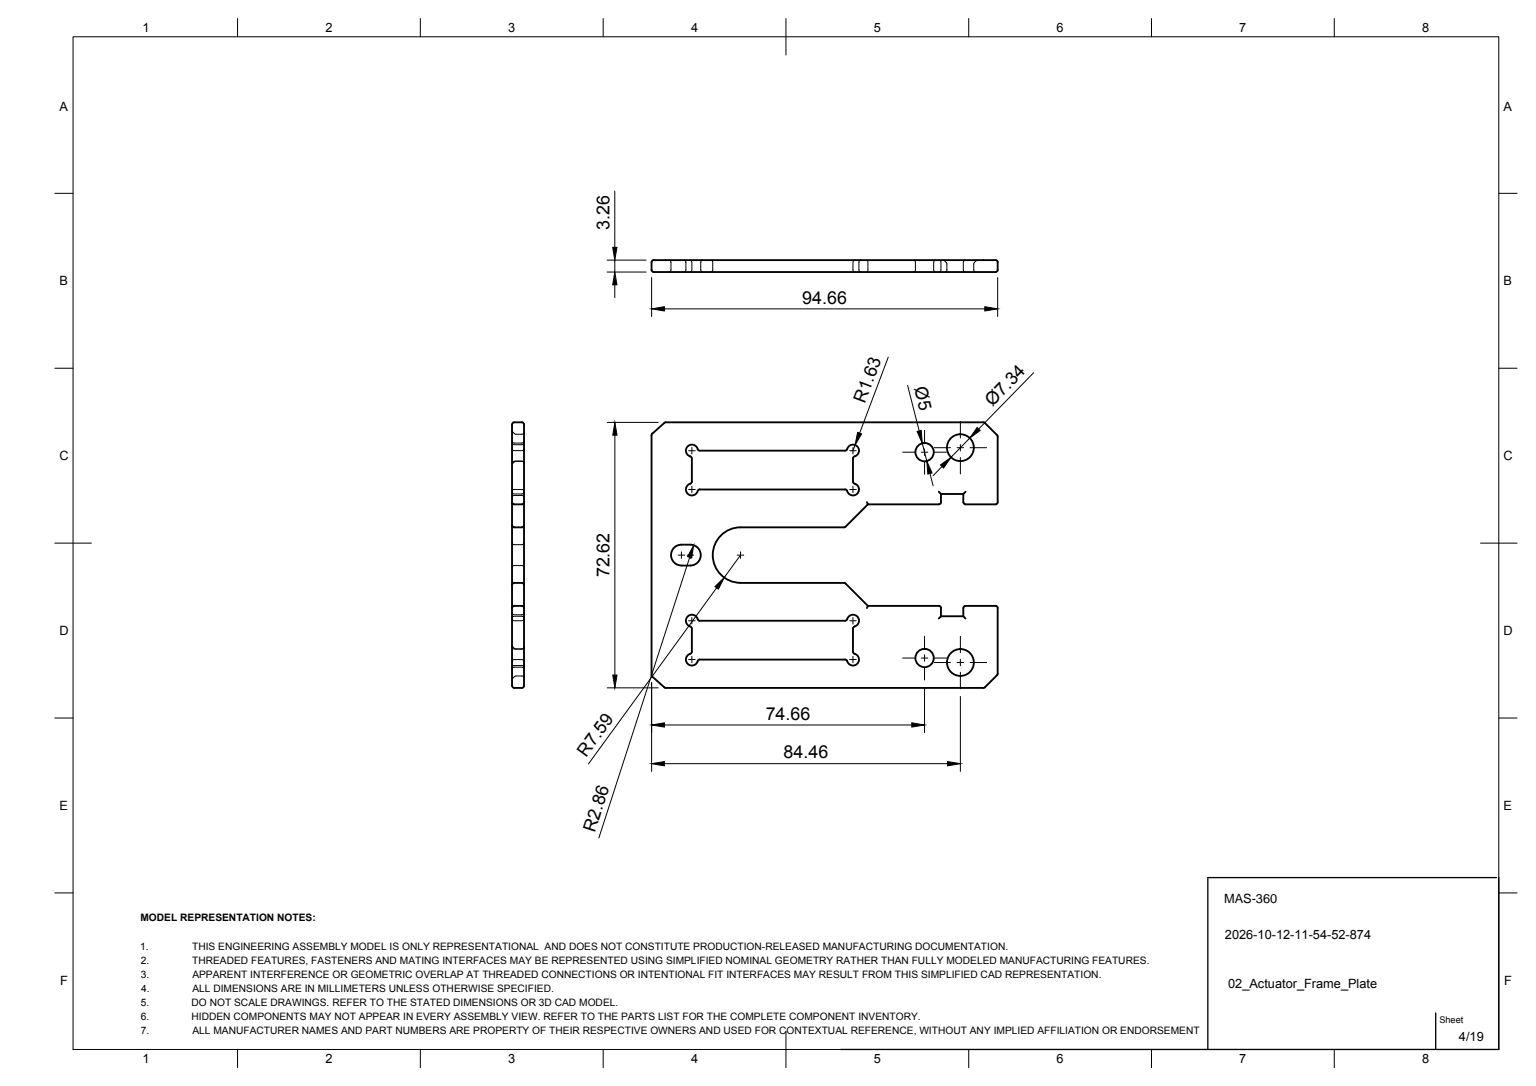
ISO-10303-21;
HEADER;
/* Generated by software containing ST-Developer
 * from STEP Tools, Inc. (www.steptools.com) 
 */

FILE_DESCRIPTION(
/* description */ (''),
/* implementation_level */ '2;1');

FILE_NAME(
/* name */ '02_Actuator_Frame_Plate.step',
/* time_stamp */ '2026-11-04T18:53:29-08:00',
/* author */ (''),
/* organization */ (''),
/* preprocessor_version */ 'ST-DEVELOPER v20.2',
/* originating_system */ 'Autodesk Translation Framework v15.17.0.0',
/* authorisation */ '');

FILE_SCHEMA (('AUTOMOTIVE_DESIGN { 1 0 10303 214 3 1 1 }'));
ENDSEC;

DATA;
#10=MECHANICAL_DESIGN_GEOMETRIC_PRESENTATION_REPRESENTATION('',(#1328),#100031);
#117=SPHERICAL_SURFACE('',#20359,0.6);
#118=SPHERICAL_SURFACE('',#20362,0.6);
#119=SPHERICAL_SURFACE('',#20376,0.6);
#120=SPHERICAL_SURFACE('',#20379,0.6);
#121=SPHERICAL_SURFACE('',#20389,0.6);
#122=SPHERICAL_SURFACE('',#20391,0.6);
#123=SPHERICAL_SURFACE('',#20401,0.6);
#124=SPHERICAL_SURFACE('',#20404,0.6);
#125=SPHERICAL_SURFACE('',#20414,0.6);
#126=SPHERICAL_SURFACE('',#20417,0.6);
#127=SPHERICAL_SURFACE('',#20430,0.6);
#128=SPHERICAL_SURFACE('',#20432,0.6);
#129=SPHERICAL_SURFACE('',#20487,0.6);
#130=SPHERICAL_SURFACE('',#20492,0.6);
#131=SPHERICAL_SURFACE('',#20504,0.6);
#132=SPHERICAL_SURFACE('',#20509,0.600000000000001);
#133=SPHERICAL_SURFACE('',#20513,0.6);
#134=SPHERICAL_SURFACE('',#20518,0.600000000000001);
#135=SPHERICAL_SURFACE('',#20523,0.600000000000001);
#136=SPHERICAL_SURFACE('',#20530,0.6);
#137=SPHERICAL_SURFACE('',#20535,0.6);
#138=SPHERICAL_SURFACE('',#20540,0.6);
#139=SPHERICAL_SURFACE('',#20545,0.6);
#140=SPHERICAL_SURFACE('',#20554,0.6);
#141=SPHERICAL_SURFACE('',#20558,0.6);
#142=SPHERICAL_SURFACE('',#20566,0.6);
#143=SPHERICAL_SURFACE('',#20577,0.6);
#144=SPHERICAL_SURFACE('',#20582,0.6);
#145=SPHERICAL_SURFACE('',#20603,0.600000000000001);
#146=SPHERICAL_SURFACE('',#20608,0.600000000000001);
#147=SPHERICAL_SURFACE('',#20613,0.600000000000001);
#148=SPHERICAL_SURFACE('',#20618,0.600000000000001);
#149=SPHERICAL_SURFACE('',#20627,0.600000000000001);
#150=SPHERICAL_SURFACE('',#20635,0.6);
#151=SPHERICAL_SURFACE('',#20640,0.6);
#152=SPHERICAL_SURFACE('',#20645,0.6);
#153=SPHERICAL_SURFACE('',#20650,0.6);
#154=SPHERICAL_SURFACE('',#20655,0.6);
#155=SPHERICAL_SURFACE('',#20660,0.6);
#156=SPHERICAL_SURFACE('',#20690,0.600000000000001);
#157=SPHERICAL_SURFACE('',#20697,0.6);
#158=SPHERICAL_SURFACE('',#20698,0.6);
#159=SPHERICAL_SURFACE('',#20704,0.6);
#160=SPHERICAL_SURFACE('',#20713,0.600000000000001);
#161=SPHERICAL_SURFACE('',#20716,0.600000000000005);
#162=SPHERICAL_SURFACE('',#20721,0.6);
#163=SPHERICAL_SURFACE('',#20729,0.6);
#164=SPHERICAL_SURFACE('',#20732,0.6);
#165=SPHERICAL_SURFACE('',#20737,0.6);
#166=SPHERICAL_SURFACE('',#20742,0.6);
#167=SPHERICAL_SURFACE('',#20749,0.6);
#168=SPHERICAL_SURFACE('',#20755,0.6);
#169=SPHERICAL_SURFACE('',#20763,0.6);
#170=SPHERICAL_SURFACE('',#20769,0.600000000000001);
#171=SPHERICAL_SURFACE('',#20779,0.600000000000001);
#172=SPHERICAL_SURFACE('',#20788,0.600000000000001);
#173=SPHERICAL_SURFACE('',#20793,0.600000000000001);
#174=SPHERICAL_SURFACE('',#20798,0.600000000000001);
#175=SPHERICAL_SURFACE('',#20810,0.6);
#176=SPHERICAL_SURFACE('',#20815,0.6);
#177=SPHERICAL_SURFACE('',#20820,0.6);
#178=SPHERICAL_SURFACE('',#20825,0.6);
#179=SPHERICAL_SURFACE('',#20830,0.6);
#180=SPHERICAL_SURFACE('',#20832,0.6);
#227=CONICAL_SURFACE('',#20353,4.08,0.785398163397448);
#228=CONICAL_SURFACE('',#20885,4.08,0.785398163397448);
#250=CIRCLE('',#20345,3.84773593128807);
#251=CIRCLE('',#20346,0.6);
#252=CIRCLE('',#20347,3.672);
#253=CIRCLE('',#20348,3.672);
#254=CIRCLE('',#20349,3.84773593128807);
#255=CIRCLE('',#20351,3.672);
#256=CIRCLE('',#20352,3.672);
#257=CIRCLE('',#20354,4.31226406871192);
#258=CIRCLE('',#20355,4.31226406871192);
#259=CIRCLE('',#20357,0.600000000000001);
#260=CIRCLE('',#20358,0.599999999999999);
#261=CIRCLE('',#20360,0.6);
#262=CIRCLE('',#20361,0.599999999999999);
#263=CIRCLE('',#20363,0.599999999999999);
#264=CIRCLE('',#20364,0.6);
#265=CIRCLE('',#20366,0.599999999999999);
#266=CIRCLE('',#20368,1.632);
#267=CIRCLE('',#20369,0.599999999999998);
#268=CIRCLE('',#20370,2.232);
#269=CIRCLE('',#20372,1.632);
#270=CIRCLE('',#20374,0.600000000000001);
#271=CIRCLE('',#20375,0.599999999999998);
#272=CIRCLE('',#20377,0.6);
#273=CIRCLE('',#20378,0.599999999999999);
#274=CIRCLE('',#20380,0.6);
#275=CIRCLE('',#20382,2.232);
#276=CIRCLE('',#20383,0.6);
#277=CIRCLE('',#20384,1.632);
#278=CIRCLE('',#20387,0.600000000000001);
#279=CIRCLE('',#20388,0.599999999999998);
#280=CIRCLE('',#20390,0.599999999999999);
#281=CIRCLE('',#20392,0.599999999999999);
#282=CIRCLE('',#20393,0.6);
#283=CIRCLE('',#20395,0.599999999999999);
#284=CIRCLE('',#20397,1.632);
#285=CIRCLE('',#20399,0.600000000000001);
#286=CIRCLE('',#20400,0.600000000000003);
#287=CIRCLE('',#20402,0.6);
#288=CIRCLE('',#20403,0.599999999999999);
#289=CIRCLE('',#20405,0.6);
#290=CIRCLE('',#20407,2.232);
#291=CIRCLE('',#20408,0.600000000000001);
#292=CIRCLE('',#20409,1.632);
#293=CIRCLE('',#20412,0.600000000000001);
#294=CIRCLE('',#20413,0.600000000000003);
#295=CIRCLE('',#20415,0.6);
#296=CIRCLE('',#20416,0.6);
#297=CIRCLE('',#20418,0.6);
#298=CIRCLE('',#20419,0.6);
#299=CIRCLE('',#20421,2.232);
#300=CIRCLE('',#20422,0.6);
#301=CIRCLE('',#20423,1.632);
#302=CIRCLE('',#20425,0.6);
#303=CIRCLE('',#20428,0.599999999999996);
#304=CIRCLE('',#20429,0.599999999999999);
#305=CIRCLE('',#20431,0.599999999999999);
#306=CIRCLE('',#20433,0.599999999999999);
#307=CIRCLE('',#20434,0.6);
#308=CIRCLE('',#20436,0.599999999999999);
#309=CIRCLE('',#20438,1.632);
#310=CIRCLE('',#20440,3.1);
#311=CIRCLE('',#20441,0.6);
#312=CIRCLE('',#20442,2.5);
#313=CIRCLE('',#20443,2.5);
#314=CIRCLE('',#20445,8.1888);
#315=CIRCLE('',#20446,4.272);
#316=CIRCLE('',#20447,3.456);
#317=CIRCLE('',#20448,3.456);
#318=CIRCLE('',#20449,2.232);
#319=CIRCLE('',#20450,2.232);
#320=CIRCLE('',#20451,2.232);
#321=CIRCLE('',#20452,2.232);
#322=CIRCLE('',#20453,3.1);
#323=CIRCLE('',#20454,2.232);
#324=CIRCLE('',#20455,2.232);
#325=CIRCLE('',#20456,2.232);
#326=CIRCLE('',#20457,2.232);
#327=CIRCLE('',#20458,4.272);
#328=CIRCLE('',#20460,2.5);
#329=CIRCLE('',#20461,2.5);
#330=CIRCLE('',#20463,0.6);
#331=CIRCLE('',#20464,3.672);
#332=CIRCLE('',#20465,3.672);
#333=CIRCLE('',#20467,3.672);
#334=CIRCLE('',#20468,3.672);
#335=CIRCLE('',#20470,0.6);
#336=CIRCLE('',#20472,0.600000000000005);
#337=CIRCLE('',#20473,0.6);
#338=CIRCLE('',#20475,0.6);
#339=CIRCLE('',#20476,2.856);
#340=CIRCLE('',#20478,0.6);
#341=CIRCLE('',#20480,2.856);
#342=CIRCLE('',#20482,2.856);
#343=CIRCLE('',#20485,0.600000000000001);
#344=CIRCLE('',#20488,0.600000000000001);
#345=CIRCLE('',#20489,0.6);
#346=CIRCLE('',#20490,0.6);
#347=CIRCLE('',#20493,0.600000000000001);
#348=CIRCLE('',#20494,0.6);
#349=CIRCLE('',#20497,0.599999999999998);
#350=CIRCLE('',#20499,0.600000000000001);
#351=CIRCLE('',#20500,1.632);
#352=CIRCLE('',#20503,0.600000000000001);
#353=CIRCLE('',#20505,0.599999999999999);
#354=CIRCLE('',#20506,0.6);
#355=CIRCLE('',#20508,0.600000000000001);
#356=CIRCLE('',#20510,0.600000000000001);
#357=CIRCLE('',#20511,0.600000000000001);
#358=CIRCLE('',#20512,0.599999999999991);
#359=CIRCLE('',#20514,0.600000000000001);
#360=CIRCLE('',#20515,0.6);
#361=CIRCLE('',#20516,0.600000000000003);
#362=CIRCLE('',#20519,0.600000000000001);
#363=CIRCLE('',#20520,0.600000000000001);
#364=CIRCLE('',#20521,0.599999999999996);
#365=CIRCLE('',#20524,0.599999999999996);
#366=CIRCLE('',#20525,0.600000000000001);
#367=CIRCLE('',#20526,0.600000000000001);
#368=CIRCLE('',#20529,0.600000000000001);
#369=CIRCLE('',#20531,0.600000000000003);
#370=CIRCLE('',#20532,0.6);
#371=CIRCLE('',#20534,0.600000000000001);
#372=CIRCLE('',#20536,0.600000000000003);
#373=CIRCLE('',#20537,0.599999999999999);
#374=CIRCLE('',#20539,0.599999999999996);
#375=CIRCLE('',#20541,0.599999999999999);
#376=CIRCLE('',#20542,0.599999999999998);
#377=CIRCLE('',#20544,0.60000000000001);
#378=CIRCLE('',#20546,0.600000000000003);
#379=CIRCLE('',#20547,0.599999999999999);
#380=CIRCLE('',#20552,0.600000000000003);
#381=CIRCLE('',#20555,0.600000000000001);
#382=CIRCLE('',#20556,0.6);
#383=CIRCLE('',#20557,0.600000000000001);
#384=CIRCLE('',#20559,0.6);
#385=CIRCLE('',#20560,0.599999999999999);
#386=CIRCLE('',#20561,0.6);
#387=CIRCLE('',#20564,0.600000000000003);
#388=CIRCLE('',#20565,1.632);
#389=CIRCLE('',#20567,0.600000000000001);
#390=CIRCLE('',#20568,0.6);
#391=CIRCLE('',#20570,0.600000000000005);
#392=CIRCLE('',#20572,1.632);
#393=CIRCLE('',#20573,0.599999999999998);
#394=CIRCLE('',#20578,0.6);
#395=CIRCLE('',#20579,0.6);
#396=CIRCLE('',#20580,0.6);
#397=CIRCLE('',#20583,0.599999999999998);
#398=CIRCLE('',#20585,2.232);
#399=CIRCLE('',#20586,0.6);
#400=CIRCLE('',#20587,1.632);
#401=CIRCLE('',#20589,0.599999999999999);
#402=CIRCLE('',#20592,0.600000000000004);
#403=CIRCLE('',#20595,0.600000000000001);
#404=CIRCLE('',#20597,0.6);
#405=CIRCLE('',#20598,2.5);
#406=CIRCLE('',#20599,2.5);
#407=CIRCLE('',#20601,2.5);
#408=CIRCLE('',#20602,2.5);
#409=CIRCLE('',#20604,0.600000000000001);
#410=CIRCLE('',#20605,0.600000000000001);
#411=CIRCLE('',#20606,0.599999999999999);
#412=CIRCLE('',#20609,0.599999999999996);
#413=CIRCLE('',#20610,0.600000000000001);
#414=CIRCLE('',#20611,0.599999999999996);
#415=CIRCLE('',#20614,0.599999999999987);
#416=CIRCLE('',#20615,0.600000000000001);
#417=CIRCLE('',#20616,0.600000000000001);
#418=CIRCLE('',#20619,0.600000000000001);
#419=CIRCLE('',#20620,0.600000000000001);
#420=CIRCLE('',#20621,0.600000000000001);
#421=CIRCLE('',#20628,0.600000000000005);
#422=CIRCLE('',#20629,0.600000000000001);
#423=CIRCLE('',#20630,0.600000000000001);
#424=CIRCLE('',#20634,0.600000000000001);
#425=CIRCLE('',#20636,0.599999999999999);
#426=CIRCLE('',#20637,0.599999999999999);
#427=CIRCLE('',#20639,0.600000000000001);
#428=CIRCLE('',#20641,0.600000000000003);
#429=CIRCLE('',#20642,0.599999999999999);
#430=CIRCLE('',#20644,0.600000000000001);
#431=CIRCLE('',#20646,0.599999999999999);
#432=CIRCLE('',#20647,0.599999999999999);
#433=CIRCLE('',#20649,0.599999999999996);
#434=CIRCLE('',#20651,0.599999999999999);
#435=CIRCLE('',#20652,0.600000000000001);
#436=CIRCLE('',#20654,0.599999999999996);
#437=CIRCLE('',#20656,0.600000000000003);
#438=CIRCLE('',#20657,0.599999999999999);
#439=CIRCLE('',#20659,0.600000000000001);
#440=CIRCLE('',#20661,0.599999999999999);
#441=CIRCLE('',#20678,3.1);
#442=CIRCLE('',#20679,0.6);
#443=CIRCLE('',#20681,8.1888);
#444=CIRCLE('',#20682,2.232);
#445=CIRCLE('',#20683,2.232);
#446=CIRCLE('',#20684,2.232);
#447=CIRCLE('',#20685,3.456);
#448=CIRCLE('',#20686,3.456);
#449=CIRCLE('',#20687,4.73652813742386);
#450=CIRCLE('',#20688,4.73652813742386);
#451=CIRCLE('',#20689,3.1);
#452=CIRCLE('',#20691,0.600000000000001);
#453=CIRCLE('',#20693,0.600000000000001);
#454=CIRCLE('',#20696,0.600000000000003);
#455=CIRCLE('',#20705,0.600000000000001);
#456=CIRCLE('',#20706,0.600000000000003);
#457=CIRCLE('',#20707,0.6);
#458=CIRCLE('',#20714,0.599999999999999);
#459=CIRCLE('',#20715,0.600000000000001);
#460=CIRCLE('',#20717,0.600000000000001);
#461=CIRCLE('',#20718,0.600000000000005);
#462=CIRCLE('',#20719,0.599999999999998);
#463=CIRCLE('',#20722,0.599999999999998);
#464=CIRCLE('',#20723,0.599999999999999);
#465=CIRCLE('',#20724,0.599999999999999);
#466=CIRCLE('',#20726,1.632);
#467=CIRCLE('',#20728,0.599999999999998);
#468=CIRCLE('',#20730,0.6);
#469=CIRCLE('',#20731,0.599999999999999);
#470=CIRCLE('',#20733,0.6);
#471=CIRCLE('',#20734,0.599999999999999);
#472=CIRCLE('',#20735,0.6);
#473=CIRCLE('',#20738,0.6);
#474=CIRCLE('',#20740,1.632);
#475=CIRCLE('',#20743,0.599999999999998);
#476=CIRCLE('',#20744,0.6);
#477=CIRCLE('',#20747,1.632);
#478=CIRCLE('',#20748,0.600000000000003);
#479=CIRCLE('',#20750,0.600000000000001);
#480=CIRCLE('',#20751,0.599999999999999);
#481=CIRCLE('',#20753,0.6);
#482=CIRCLE('',#20754,1.632);
#483=CIRCLE('',#20756,0.6);
#484=CIRCLE('',#20757,0.599999999999999);
#485=CIRCLE('',#20758,0.6);
#486=CIRCLE('',#20762,0.600000000000003);
#487=CIRCLE('',#20764,0.599999999999999);
#488=CIRCLE('',#20768,0.599999999999999);
#489=CIRCLE('',#20770,0.600000000000001);
#490=CIRCLE('',#20771,0.600000000000001);
#491=CIRCLE('',#20772,0.599999999999999);
#492=CIRCLE('',#20774,0.600000000000001);
#493=CIRCLE('',#20775,7.5888);
#494=CIRCLE('',#20780,0.600000000000001);
#495=CIRCLE('',#20781,0.600000000000001);
#496=CIRCLE('',#20782,0.600000000000001);
#497=CIRCLE('',#20789,0.600000000000001);
#498=CIRCLE('',#20790,0.600000000000001);
#499=CIRCLE('',#20791,0.600000000000001);
#500=CIRCLE('',#20794,0.600000000000001);
#501=CIRCLE('',#20795,0.600000000000001);
#502=CIRCLE('',#20796,0.599999999999996);
#503=CIRCLE('',#20799,0.599999999999996);
#504=CIRCLE('',#20800,0.600000000000001);
#505=CIRCLE('',#20801,0.599999999999999);
#506=CIRCLE('',#20805,0.599999999999999);
#507=CIRCLE('',#20807,0.600000000000001);
#508=CIRCLE('',#20809,0.599999999999996);
#509=CIRCLE('',#20811,0.599999999999999);
#510=CIRCLE('',#20812,0.599999999999999);
#511=CIRCLE('',#20814,0.600000000000001);
#512=CIRCLE('',#20816,0.599999999999999);
#513=CIRCLE('',#20817,0.600000000000003);
#514=CIRCLE('',#20819,0.600000000000001);
#515=CIRCLE('',#20821,0.599999999999999);
#516=CIRCLE('',#20822,0.599999999999999);
#517=CIRCLE('',#20824,0.599999999999999);
#518=CIRCLE('',#20826,0.599999999999999);
#519=CIRCLE('',#20827,0.6);
#520=CIRCLE('',#20829,0.600000000000001);
#521=CIRCLE('',#20831,0.599999999999999);
#522=CIRCLE('',#20833,0.6);
#523=CIRCLE('',#20835,0.600000000000001);
#524=CIRCLE('',#20855,0.600000000000001);
#525=CIRCLE('',#20857,7.5888);
#526=CIRCLE('',#20863,1.632);
#527=CIRCLE('',#20868,0.6);
#528=CIRCLE('',#20870,0.600000000000001);
#529=CIRCLE('',#20871,0.6);
#530=CIRCLE('',#20873,0.6);
#531=CIRCLE('',#20874,2.856);
#532=CIRCLE('',#20876,0.6);
#533=CIRCLE('',#20880,0.6);
#534=CIRCLE('',#20882,4.31226406871192);
#535=CIRCLE('',#20883,0.6);
#536=CIRCLE('',#20884,4.31226406871192);
#537=CIRCLE('',#20886,3.84773593128807);
#538=CIRCLE('',#20887,3.84773593128807);
#539=CIRCLE('',#20889,0.6);
#1183=TOROIDAL_SURFACE('',#20344,4.272,0.6);
#1184=TOROIDAL_SURFACE('',#20367,2.232,0.6);
#1185=TOROIDAL_SURFACE('',#20381,2.232,0.6);
#1186=TOROIDAL_SURFACE('',#20406,2.232,0.6);
#1187=TOROIDAL_SURFACE('',#20420,2.232,0.6);
#1188=TOROIDAL_SURFACE('',#20439,3.1,0.6);
#1189=TOROIDAL_SURFACE('',#20462,4.272,0.6);
#1190=TOROIDAL_SURFACE('',#20469,4.272,0.6);
#1191=TOROIDAL_SURFACE('',#20474,3.456,0.6);
#1192=TOROIDAL_SURFACE('',#20479,3.456,0.6);
#1193=TOROIDAL_SURFACE('',#20486,2.232,0.6);
#1194=TOROIDAL_SURFACE('',#20498,2.232,0.6);
#1195=TOROIDAL_SURFACE('',#20563,2.232,0.6);
#1196=TOROIDAL_SURFACE('',#20571,2.232,0.6);
#1197=TOROIDAL_SURFACE('',#20575,2.232,0.6);
#1198=TOROIDAL_SURFACE('',#20581,2.232,0.6);
#1199=TOROIDAL_SURFACE('',#20584,2.232,0.6);
#1200=TOROIDAL_SURFACE('',#20596,3.1,0.6);
#1201=TOROIDAL_SURFACE('',#20677,3.1,0.6);
#1202=TOROIDAL_SURFACE('',#20725,2.232,0.6);
#1203=TOROIDAL_SURFACE('',#20741,2.232,0.6);
#1204=TOROIDAL_SURFACE('',#20746,2.232,0.6);
#1205=TOROIDAL_SURFACE('',#20752,2.232,0.6);
#1206=TOROIDAL_SURFACE('',#20773,8.1888,0.6);
#1207=TOROIDAL_SURFACE('',#20856,8.1888,0.6);
#1208=TOROIDAL_SURFACE('',#20862,2.232,0.6);
#1209=TOROIDAL_SURFACE('',#20867,3.1,0.6);
#1210=TOROIDAL_SURFACE('',#20872,3.456,0.6);
#1211=TOROIDAL_SURFACE('',#20877,3.456,0.6);
#1212=TOROIDAL_SURFACE('',#20879,4.73652813742386,0.6);
#1213=TOROIDAL_SURFACE('',#20881,4.73652813742386,0.6);
#1214=TOROIDAL_SURFACE('',#20888,4.272,0.6);
#1292=SHAPE_REPRESENTATION_RELATIONSHIP('SRR','None',#100102,#1310);
#1310=ADVANCED_BREP_SHAPE_REPRESENTATION('',(#1346),#100014);
#1328=STYLED_ITEM('',(#100201),#1346);
#1346=MANIFOLD_SOLID_BREP('Body1',#20118);
#1364=PLANE('',#20385);
#1365=PLANE('',#20410);
#1366=PLANE('',#20426);
#1367=PLANE('',#20444);
#1368=PLANE('',#20483);
#1369=PLANE('',#20495);
#1370=PLANE('',#20548);
#1371=PLANE('',#20549);
#1372=PLANE('',#20553);
#1373=PLANE('',#20590);
#1374=PLANE('',#20662);
#1375=PLANE('',#20665);
#1376=PLANE('',#20669);
#1377=PLANE('',#20670);
#1378=PLANE('',#20671);
#1379=PLANE('',#20676);
#1380=PLANE('',#20680);
#1381=PLANE('',#20700);
#1382=PLANE('',#20709);
#1383=PLANE('',#20710);
#1384=PLANE('',#20711);
#1385=PLANE('',#20765);
#1386=PLANE('',#20838);
#1387=PLANE('',#20839);
#1388=PLANE('',#20843);
#1389=PLANE('',#20844);
#1390=PLANE('',#20845);
#1391=PLANE('',#20848);
#1392=PLANE('',#20850);
#1393=PLANE('',#20852);
#1394=PLANE('',#20858);
#1395=PLANE('',#20860);
#1396=PLANE('',#20866);
#1397=PLANE('',#20890);
#1398=PLANE('',#20891);
#1703=FACE_BOUND('',#6316,.T.);
#1704=FACE_BOUND('',#6317,.T.);
#1705=FACE_BOUND('',#6318,.T.);
#1706=FACE_BOUND('',#6319,.T.);
#1707=FACE_BOUND('',#6320,.T.);
#1708=FACE_BOUND('',#6321,.T.);
#1709=FACE_BOUND('',#6322,.T.);
#1710=FACE_BOUND('',#6424,.T.);
#1711=FACE_BOUND('',#6425,.T.);
#1712=FACE_BOUND('',#6426,.T.);
#1713=FACE_BOUND('',#6427,.T.);
#1714=FACE_BOUND('',#6428,.T.);
#1715=FACE_BOUND('',#6429,.T.);
#1716=FACE_BOUND('',#6430,.T.);
#1813=ELLIPSE('',#20502,0.649435320175436,0.6);
#1814=ELLIPSE('',#20624,0.848528137423857,0.6);
#1815=ELLIPSE('',#20626,0.848528137423857,0.6);
#1816=ELLIPSE('',#20668,0.848528137423857,0.6);
#1817=ELLIPSE('',#20673,0.848528137423857,0.6);
#1818=ELLIPSE('',#20675,0.649435320175435,0.6);
#1819=ELLIPSE('',#20778,0.649435320175437,0.6);
#1820=ELLIPSE('',#20785,0.848528137423857,0.6);
#1821=ELLIPSE('',#20787,0.848528137423857,0.6);
#1822=ELLIPSE('',#20837,0.649435320175436,0.6);
#1823=ELLIPSE('',#20842,0.848528137423857,0.6);
#1824=ELLIPSE('',#20847,0.848528137423857,0.6);
#2070=LINE('',#59081,#3357);
#2071=LINE('',#59084,#3358);
#2072=LINE('',#59093,#3359);
#2073=LINE('',#59096,#3360);
#2074=LINE('',#59107,#3361);
#2075=LINE('',#59110,#3362);
#2076=LINE('',#59120,#3363);
#2077=LINE('',#59125,#3364);
#2078=LINE('',#59128,#3365);
#2079=LINE('',#59142,#3366);
#2080=LINE('',#59147,#3367);
#2081=LINE('',#59150,#3368);
#2082=LINE('',#59159,#3369);
#2083=LINE('',#59162,#3370);
#2084=LINE('',#59169,#3371);
#2085=LINE('',#59172,#3372);
#2086=LINE('',#59186,#3373);
#2087=LINE('',#59192,#3374);
#2088=LINE('',#59195,#3375);
#2089=LINE('',#59212,#3376);
#2090=LINE('',#59215,#3377);
#2091=LINE('',#59218,#3378);
#2092=LINE('',#59219,#3379);
#2093=LINE('',#59224,#3380);
#2094=LINE('',#59227,#3381);
#2095=LINE('',#59236,#3382);
#2096=LINE('',#59239,#3383);
#2097=LINE('',#59253,#3384);
#2098=LINE('',#59255,#3385);
#2099=LINE('',#59257,#3386);
#2100=LINE('',#59259,#3387);
#2101=LINE('',#59261,#3388);
#2102=LINE('',#59263,#3389);
#2103=LINE('',#59265,#3390);
#2104=LINE('',#59267,#3391);
#2105=LINE('',#59269,#3392);
#2106=LINE('',#59271,#3393);
#2107=LINE('',#59273,#3394);
#2108=LINE('',#59275,#3395);
#2109=LINE('',#59277,#3396);
#2110=LINE('',#59279,#3397);
#2111=LINE('',#59281,#3398);
#2112=LINE('',#59283,#3399);
#2113=LINE('',#59285,#3400);
#2114=LINE('',#59287,#3401);
#2115=LINE('',#59289,#3402);
#2116=LINE('',#59291,#3403);
#2117=LINE('',#59293,#3404);
#2118=LINE('',#59295,#3405);
#2119=LINE('',#59298,#3406);
#2120=LINE('',#59303,#3407);
#2121=LINE('',#59307,#3408);
#2122=LINE('',#59310,#3409);
#2123=LINE('',#59314,#3410);
#2124=LINE('',#59318,#3411);
#2125=LINE('',#59321,#3412);
#2126=LINE('',#59329,#3413);
#2127=LINE('',#59331,#3414);
#2128=LINE('',#59333,#3415);
#2129=LINE('',#59336,#3416);
#2130=LINE('',#59341,#3417);
#2131=LINE('',#59353,#3418);
#2132=LINE('',#59363,#3419);
#2133=LINE('',#59372,#3420);
#2134=LINE('',#59377,#3421);
#2135=LINE('',#59380,#3422);
#2136=LINE('',#59383,#3423);
#2137=LINE('',#59384,#3424);
#2138=LINE('',#59387,#3425);
#2139=LINE('',#59401,#3426);
#2140=LINE('',#59404,#3427);
#2141=LINE('',#59415,#3428);
#2142=LINE('',#59423,#3429);
#2143=LINE('',#59437,#3430);
#2144=LINE('',#59445,#3431);
#2145=LINE('',#59453,#3432);
#2146=LINE('',#59457,#3433);
#2147=LINE('',#59466,#3434);
#2148=LINE('',#59467,#3435);
#2149=LINE('',#59476,#3436);
#2150=LINE('',#59477,#3437);
#2151=LINE('',#59486,#3438);
#2152=LINE('',#59487,#3439);
#2153=LINE('',#59493,#3440);
#2154=LINE('',#59495,#3441);
#2155=LINE('',#59497,#3442);
#2156=LINE('',#59500,#3443);
#2157=LINE('',#59503,#3444);
#2158=LINE('',#59505,#3445);
#2159=LINE('',#59520,#3446);
#2160=LINE('',#59521,#3447);
#2161=LINE('',#59533,#3448);
#2162=LINE('',#59557,#3449);
#2163=LINE('',#59559,#3450);
#2164=LINE('',#59561,#3451);
#2165=LINE('',#59563,#3452);
#2166=LINE('',#59568,#3453);
#2167=LINE('',#59578,#3454);
#2168=LINE('',#59589,#3455);
#2169=LINE('',#59597,#3456);
#2170=LINE('',#59605,#3457);
#2171=LINE('',#59613,#3458);
#2172=LINE('',#59616,#3459);
#2173=LINE('',#59621,#3460);
#2174=LINE('',#59629,#3461);
#2175=LINE('',#59631,#3462);
#2176=LINE('',#59636,#3463);
#2177=LINE('',#59637,#3464);
#2178=LINE('',#59646,#3465);
#2179=LINE('',#59647,#3466);
#2180=LINE('',#59656,#3467);
#2181=LINE('',#59657,#3468);
#2182=LINE('',#59666,#3469);
#2183=LINE('',#59667,#3470);
#2184=LINE('',#59676,#3471);
#2185=LINE('',#59677,#3472);
#2186=LINE('',#59684,#3473);
#2187=LINE('',#59689,#3474);
#2188=LINE('',#59691,#3475);
#2189=LINE('',#59692,#3476);
#2190=LINE('',#59694,#3477);
#2191=LINE('',#59696,#3478);
#2192=LINE('',#59698,#3479);
#2193=LINE('',#59701,#3480);
#2194=LINE('',#59704,#3481);
#2195=LINE('',#59706,#3482);
#2196=LINE('',#59709,#3483);
#2197=LINE('',#59710,#3484);
#2198=LINE('',#59712,#3485);
#2199=LINE('',#59715,#3486);
#2200=LINE('',#59719,#3487);
#2201=LINE('',#59722,#3488);
#2202=LINE('',#59724,#3489);
#2203=LINE('',#59731,#3490);
#2204=LINE('',#59733,#3491);
#2205=LINE('',#59737,#3492);
#2206=LINE('',#59739,#3493);
#2207=LINE('',#59741,#3494);
#2208=LINE('',#59743,#3495);
#2209=LINE('',#59745,#3496);
#2210=LINE('',#59747,#3497);
#2211=LINE('',#59749,#3498);
#2212=LINE('',#59751,#3499);
#2213=LINE('',#59753,#3500);
#2214=LINE('',#59754,#3501);
#2215=LINE('',#59755,#3502);
#2216=LINE('',#59756,#3503);
#2217=LINE('',#59757,#3504);
#2218=LINE('',#59761,#3505);
#2219=LINE('',#59765,#3506);
#2220=LINE('',#59769,#3507);
#2221=LINE('',#59773,#3508);
#2222=LINE('',#59777,#3509);
#2223=LINE('',#59787,#3510);
#2224=LINE('',#59789,#3511);
#2225=LINE('',#59791,#3512);
#2226=LINE('',#59793,#3513);
#2227=LINE('',#59800,#3514);
#2228=LINE('',#59809,#3515);
#2229=LINE('',#59813,#3516);
#2230=LINE('',#59815,#3517);
#2231=LINE('',#59827,#3518);
#2232=LINE('',#59840,#3519);
#2233=LINE('',#59841,#3520);
#2234=LINE('',#59852,#3521);
#2235=LINE('',#59853,#3522);
#2236=LINE('',#59864,#3523);
#2237=LINE('',#59884,#3524);
#2238=LINE('',#59885,#3525);
#2239=LINE('',#59887,#3526);
#2240=LINE('',#59889,#3527);
#2241=LINE('',#59892,#3528);
#2242=LINE('',#59896,#3529);
#2243=LINE('',#59901,#3530);
#2244=LINE('',#59913,#3531);
#2245=LINE('',#59916,#3532);
#2246=LINE('',#59925,#3533);
#2247=LINE('',#59928,#3534);
#2248=LINE('',#59933,#3535);
#2249=LINE('',#59941,#3536);
#2250=LINE('',#59949,#3537);
#2251=LINE('',#59957,#3538);
#2252=LINE('',#59959,#3539);
#2253=LINE('',#59964,#3540);
#2254=LINE('',#59965,#3541);
#2255=LINE('',#59968,#3542);
#2256=LINE('',#59973,#3543);
#2257=LINE('',#59974,#3544);
#2258=LINE('',#59982,#3545);
#2259=LINE('',#59983,#3546);
#2260=LINE('',#59991,#3547);
#2261=LINE('',#59992,#3548);
#2262=LINE('',#60000,#3549);
#2263=LINE('',#60001,#3550);
#2264=LINE('',#60007,#3551);
#2265=LINE('',#60009,#3552);
#2266=LINE('',#60017,#3553);
#2267=LINE('',#60020,#3554);
#2268=LINE('',#60023,#3555);
#2269=LINE('',#60025,#3556);
#2270=LINE('',#60029,#3557);
#2271=LINE('',#60032,#3558);
#2272=LINE('',#60035,#3559);
#2273=LINE('',#60036,#3560);
#2274=LINE('',#60038,#3561);
#2275=LINE('',#60042,#3562);
#2276=LINE('',#60045,#3563);
#2277=LINE('',#60051,#3564);
#2278=LINE('',#60056,#3565);
#2279=LINE('',#60058,#3566);
#2280=LINE('',#60064,#3567);
#2281=LINE('',#60078,#3568);
#2282=LINE('',#60081,#3569);
#2283=LINE('',#60095,#3570);
#3357=VECTOR('',#22653,3.672);
#3358=VECTOR('',#22656,4.08);
#3359=VECTOR('',#22665,10.);
#3360=VECTOR('',#22668,10.);
#3361=VECTOR('',#22683,10.);
#3362=VECTOR('',#22686,10.);
#3363=VECTOR('',#22699,10.);
#3364=VECTOR('',#22704,10.);
#3365=VECTOR('',#22707,10.);
#3366=VECTOR('',#22728,10.);
#3367=VECTOR('',#22733,10.);
#3368=VECTOR('',#22736,10.);
#3369=VECTOR('',#22749,10.);
#3370=VECTOR('',#22752,10.);
#3371=VECTOR('',#22761,10.);
#3372=VECTOR('',#22764,10.);
#3373=VECTOR('',#22785,10.);
#3374=VECTOR('',#22790,10.);
#3375=VECTOR('',#22793,10.);
#3376=VECTOR('',#22816,10.);
#3377=VECTOR('',#22819,10.);
#3378=VECTOR('',#22822,10.);
#3379=VECTOR('',#22823,10.);
#3380=VECTOR('',#22828,10.);
#3381=VECTOR('',#22831,10.);
#3382=VECTOR('',#22844,10.);
#3383=VECTOR('',#22847,10.);
#3384=VECTOR('',#22864,10.);
#3385=VECTOR('',#22865,10.);
#3386=VECTOR('',#22866,10.);
#3387=VECTOR('',#22867,10.);
#3388=VECTOR('',#22868,10.);
#3389=VECTOR('',#22869,10.);
#3390=VECTOR('',#22870,10.);
#3391=VECTOR('',#22871,10.);
#3392=VECTOR('',#22872,10.);
#3393=VECTOR('',#22873,10.);
#3394=VECTOR('',#22874,10.);
#3395=VECTOR('',#22875,10.);
#3396=VECTOR('',#22876,10.);
#3397=VECTOR('',#22877,10.);
#3398=VECTOR('',#22878,10.);
#3399=VECTOR('',#22879,10.);
#3400=VECTOR('',#22880,10.);
#3401=VECTOR('',#22881,10.);
#3402=VECTOR('',#22882,10.);
#3403=VECTOR('',#22883,10.);
#3404=VECTOR('',#22884,10.);
#3405=VECTOR('',#22885,10.);
#3406=VECTOR('',#22888,10.);
#3407=VECTOR('',#22891,10.);
#3408=VECTOR('',#22894,10.);
#3409=VECTOR('',#22897,10.);
#3410=VECTOR('',#22900,10.);
#3411=VECTOR('',#22903,10.);
#3412=VECTOR('',#22906,10.);
#3413=VECTOR('',#22913,10.);
#3414=VECTOR('',#22916,10.);
#3415=VECTOR('',#22919,10.);
#3416=VECTOR('',#22922,10.);
#3417=VECTOR('',#22927,2.5);
#3418=VECTOR('',#22942,3.672);
#3419=VECTOR('',#22955,10.);
#3420=VECTOR('',#22968,10.);
#3421=VECTOR('',#22975,10.);
#3422=VECTOR('',#22978,10.);
#3423=VECTOR('',#22981,10.);
#3424=VECTOR('',#22982,10.);
#3425=VECTOR('',#22985,10.);
#3426=VECTOR('',#23008,10.);
#3427=VECTOR('',#23011,10.);
#3428=VECTOR('',#23026,10.);
#3429=VECTOR('',#23037,10.);
#3430=VECTOR('',#23056,10.);
#3431=VECTOR('',#23067,10.);
#3432=VECTOR('',#23078,10.);
#3433=VECTOR('',#23083,10.);
#3434=VECTOR('',#23094,10.);
#3435=VECTOR('',#23095,10.);
#3436=VECTOR('',#23106,10.);
#3437=VECTOR('',#23107,10.);
#3438=VECTOR('',#23118,10.);
#3439=VECTOR('',#23119,10.);
#3440=VECTOR('',#23128,10.);
#3441=VECTOR('',#23131,10.);
#3442=VECTOR('',#23134,10.);
#3443=VECTOR('',#23137,10.);
#3444=VECTOR('',#23140,10.);
#3445=VECTOR('',#23143,10.);
#3446=VECTOR('',#23162,10.);
#3447=VECTOR('',#23163,10.);
#3448=VECTOR('',#23180,10.);
#3449=VECTOR('',#23217,10.);
#3450=VECTOR('',#23220,10.);
#3451=VECTOR('',#23223,10.);
#3452=VECTOR('',#23226,10.);
#3453=VECTOR('',#23233,10.);
#3454=VECTOR('',#23246,2.5);
#3455=VECTOR('',#23261,10.);
#3456=VECTOR('',#23272,10.);
#3457=VECTOR('',#23283,10.);
#3458=VECTOR('',#23294,10.);
#3459=VECTOR('',#23297,10.);
#3460=VECTOR('',#23304,10.);
#3461=VECTOR('',#23315,10.);
#3462=VECTOR('',#23318,10.);
#3463=VECTOR('',#23323,10.);
#3464=VECTOR('',#23324,10.);
#3465=VECTOR('',#23335,10.);
#3466=VECTOR('',#23336,10.);
#3467=VECTOR('',#23347,10.);
#3468=VECTOR('',#23348,10.);
#3469=VECTOR('',#23359,10.);
#3470=VECTOR('',#23360,10.);
#3471=VECTOR('',#23371,10.);
#3472=VECTOR('',#23372,10.);
#3473=VECTOR('',#23381,10.);
#3474=VECTOR('',#23390,10.);
#3475=VECTOR('',#23393,10.);
#3476=VECTOR('',#23394,10.);
#3477=VECTOR('',#23397,10.);
#3478=VECTOR('',#23400,10.);
#3479=VECTOR('',#23403,10.);
#3480=VECTOR('',#23406,10.);
#3481=VECTOR('',#23409,10.);
#3482=VECTOR('',#23412,10.);
#3483=VECTOR('',#23415,10.);
#3484=VECTOR('',#23416,10.);
#3485=VECTOR('',#23419,10.);
#3486=VECTOR('',#23422,10.);
#3487=VECTOR('',#23427,10.);
#3488=VECTOR('',#23430,10.);
#3489=VECTOR('',#23433,10.);
#3490=VECTOR('',#23442,10.);
#3491=VECTOR('',#23443,10.);
#3492=VECTOR('',#23446,10.);
#3493=VECTOR('',#23447,10.);
#3494=VECTOR('',#23448,10.);
#3495=VECTOR('',#23449,10.);
#3496=VECTOR('',#23450,10.);
#3497=VECTOR('',#23451,10.);
#3498=VECTOR('',#23452,10.);
#3499=VECTOR('',#23453,10.);
#3500=VECTOR('',#23454,10.);
#3501=VECTOR('',#23455,10.);
#3502=VECTOR('',#23456,10.);
#3503=VECTOR('',#23457,10.);
#3504=VECTOR('',#23458,10.);
#3505=VECTOR('',#23461,10.);
#3506=VECTOR('',#23464,10.);
#3507=VECTOR('',#23467,10.);
#3508=VECTOR('',#23470,10.);
#3509=VECTOR('',#23475,10.);
#3510=VECTOR('',#23488,10.);
#3511=VECTOR('',#23491,10.);
#3512=VECTOR('',#23494,10.);
#3513=VECTOR('',#23497,10.);
#3514=VECTOR('',#23510,10.);
#3515=VECTOR('',#23523,10.);
#3516=VECTOR('',#23530,10.);
#3517=VECTOR('',#23533,10.);
#3518=VECTOR('',#23550,10.);
#3519=VECTOR('',#23567,10.);
#3520=VECTOR('',#23568,10.);
#3521=VECTOR('',#23585,10.);
#3522=VECTOR('',#23586,10.);
#3523=VECTOR('',#23605,10.);
#3524=VECTOR('',#23634,10.);
#3525=VECTOR('',#23635,10.);
#3526=VECTOR('',#23638,10.);
#3527=VECTOR('',#23641,10.);
#3528=VECTOR('',#23644,10.);
#3529=VECTOR('',#23651,10.);
#3530=VECTOR('',#23658,10.);
#3531=VECTOR('',#23675,10.);
#3532=VECTOR('',#23678,10.);
#3533=VECTOR('',#23691,10.);
#3534=VECTOR('',#23694,10.);
#3535=VECTOR('',#23701,10.);
#3536=VECTOR('',#23712,10.);
#3537=VECTOR('',#23723,10.);
#3538=VECTOR('',#23734,10.);
#3539=VECTOR('',#23737,10.);
#3540=VECTOR('',#23742,10.);
#3541=VECTOR('',#23743,10.);
#3542=VECTOR('',#23748,10.);
#3543=VECTOR('',#23753,10.);
#3544=VECTOR('',#23754,10.);
#3545=VECTOR('',#23765,10.);
#3546=VECTOR('',#23766,10.);
#3547=VECTOR('',#23777,10.);
#3548=VECTOR('',#23778,10.);
#3549=VECTOR('',#23789,10.);
#3550=VECTOR('',#23790,10.);
#3551=VECTOR('',#23799,10.);
#3552=VECTOR('',#23802,10.);
#3553=VECTOR('',#23815,10.);
#3554=VECTOR('',#23818,10.);
#3555=VECTOR('',#23823,10.);
#3556=VECTOR('',#23826,10.);
#3557=VECTOR('',#23831,10.);
#3558=VECTOR('',#23836,10.);
#3559=VECTOR('',#23839,10.);
#3560=VECTOR('',#23840,10.);
#3561=VECTOR('',#23843,10.);
#3562=VECTOR('',#23850,10.);
#3563=VECTOR('',#23855,10.);
#3564=VECTOR('',#23864,10.);
#3565=VECTOR('',#23873,10.);
#3566=VECTOR('',#23876,10.);
#3567=VECTOR('',#23887,10.);
#3568=VECTOR('',#23912,10.);
#3569=VECTOR('',#23917,10.);
#3570=VECTOR('',#23936,4.08);
#4558=CYLINDRICAL_SURFACE('',#20350,3.672);
#4559=CYLINDRICAL_SURFACE('',#20356,0.6);
#4560=CYLINDRICAL_SURFACE('',#20365,0.6);
#4561=CYLINDRICAL_SURFACE('',#20371,1.632);
#4562=CYLINDRICAL_SURFACE('',#20373,0.6);
#4563=CYLINDRICAL_SURFACE('',#20386,0.6);
#4564=CYLINDRICAL_SURFACE('',#20394,0.6);
#4565=CYLINDRICAL_SURFACE('',#20396,1.632);
#4566=CYLINDRICAL_SURFACE('',#20398,0.6);
#4567=CYLINDRICAL_SURFACE('',#20411,0.6);
#4568=CYLINDRICAL_SURFACE('',#20424,0.6);
#4569=CYLINDRICAL_SURFACE('',#20427,0.6);
#4570=CYLINDRICAL_SURFACE('',#20435,0.6);
#4571=CYLINDRICAL_SURFACE('',#20437,1.632);
#4572=CYLINDRICAL_SURFACE('',#20459,2.5);
#4573=CYLINDRICAL_SURFACE('',#20466,3.672);
#4574=CYLINDRICAL_SURFACE('',#20471,0.6);
#4575=CYLINDRICAL_SURFACE('',#20477,0.6);
#4576=CYLINDRICAL_SURFACE('',#20481,2.856);
#4577=CYLINDRICAL_SURFACE('',#20484,0.6);
#4578=CYLINDRICAL_SURFACE('',#20491,0.6);
#4579=CYLINDRICAL_SURFACE('',#20496,0.6);
#4580=CYLINDRICAL_SURFACE('',#20501,0.6);
#4581=CYLINDRICAL_SURFACE('',#20507,0.6);
#4582=CYLINDRICAL_SURFACE('',#20517,0.6);
#4583=CYLINDRICAL_SURFACE('',#20522,0.6);
#4584=CYLINDRICAL_SURFACE('',#20527,0.6);
#4585=CYLINDRICAL_SURFACE('',#20528,0.6);
#4586=CYLINDRICAL_SURFACE('',#20533,0.6);
#4587=CYLINDRICAL_SURFACE('',#20538,0.6);
#4588=CYLINDRICAL_SURFACE('',#20543,0.6);
#4589=CYLINDRICAL_SURFACE('',#20550,0.6);
#4590=CYLINDRICAL_SURFACE('',#20551,0.6);
#4591=CYLINDRICAL_SURFACE('',#20562,0.6);
#4592=CYLINDRICAL_SURFACE('',#20569,0.6);
#4593=CYLINDRICAL_SURFACE('',#20574,0.6);
#4594=CYLINDRICAL_SURFACE('',#20576,0.6);
#4595=CYLINDRICAL_SURFACE('',#20588,0.6);
#4596=CYLINDRICAL_SURFACE('',#20591,0.6);
#4597=CYLINDRICAL_SURFACE('',#20593,1.632);
#4598=CYLINDRICAL_SURFACE('',#20594,0.6);
#4599=CYLINDRICAL_SURFACE('',#20600,2.5);
#4600=CYLINDRICAL_SURFACE('',#20607,0.6);
#4601=CYLINDRICAL_SURFACE('',#20612,0.6);
#4602=CYLINDRICAL_SURFACE('',#20617,0.6);
#4603=CYLINDRICAL_SURFACE('',#20622,0.6);
#4604=CYLINDRICAL_SURFACE('',#20623,0.6);
#4605=CYLINDRICAL_SURFACE('',#20625,0.6);
#4606=CYLINDRICAL_SURFACE('',#20631,0.6);
#4607=CYLINDRICAL_SURFACE('',#20632,0.6);
#4608=CYLINDRICAL_SURFACE('',#20633,0.6);
#4609=CYLINDRICAL_SURFACE('',#20638,0.6);
#4610=CYLINDRICAL_SURFACE('',#20643,0.6);
#4611=CYLINDRICAL_SURFACE('',#20648,0.6);
#4612=CYLINDRICAL_SURFACE('',#20653,0.6);
#4613=CYLINDRICAL_SURFACE('',#20658,0.6);
#4614=CYLINDRICAL_SURFACE('',#20663,0.6);
#4615=CYLINDRICAL_SURFACE('',#20664,0.6);
#4616=CYLINDRICAL_SURFACE('',#20666,0.6);
#4617=CYLINDRICAL_SURFACE('',#20667,0.6);
#4618=CYLINDRICAL_SURFACE('',#20672,0.6);
#4619=CYLINDRICAL_SURFACE('',#20674,0.6);
#4620=CYLINDRICAL_SURFACE('',#20692,0.6);
#4621=CYLINDRICAL_SURFACE('',#20694,0.6);
#4622=CYLINDRICAL_SURFACE('',#20695,0.6);
#4623=CYLINDRICAL_SURFACE('',#20699,1.632);
#4624=CYLINDRICAL_SURFACE('',#20701,0.6);
#4625=CYLINDRICAL_SURFACE('',#20702,0.6);
#4626=CYLINDRICAL_SURFACE('',#20703,0.6);
#4627=CYLINDRICAL_SURFACE('',#20708,0.6);
#4628=CYLINDRICAL_SURFACE('',#20712,0.6);
#4629=CYLINDRICAL_SURFACE('',#20720,0.6);
#4630=CYLINDRICAL_SURFACE('',#20727,0.6);
#4631=CYLINDRICAL_SURFACE('',#20736,0.6);
#4632=CYLINDRICAL_SURFACE('',#20739,1.632);
#4633=CYLINDRICAL_SURFACE('',#20745,0.6);
#4634=CYLINDRICAL_SURFACE('',#20759,0.6);
#4635=CYLINDRICAL_SURFACE('',#20760,0.6);
#4636=CYLINDRICAL_SURFACE('',#20761,0.6);
#4637=CYLINDRICAL_SURFACE('',#20766,1.632);
#4638=CYLINDRICAL_SURFACE('',#20767,0.6);
#4639=CYLINDRICAL_SURFACE('',#20776,0.6);
#4640=CYLINDRICAL_SURFACE('',#20777,0.6);
#4641=CYLINDRICAL_SURFACE('',#20783,0.6);
#4642=CYLINDRICAL_SURFACE('',#20784,0.6);
#4643=CYLINDRICAL_SURFACE('',#20786,0.6);
#4644=CYLINDRICAL_SURFACE('',#20792,0.6);
#4645=CYLINDRICAL_SURFACE('',#20797,0.6);
#4646=CYLINDRICAL_SURFACE('',#20802,0.6);
#4647=CYLINDRICAL_SURFACE('',#20803,0.6);
#4648=CYLINDRICAL_SURFACE('',#20804,0.6);
#4649=CYLINDRICAL_SURFACE('',#20806,0.6);
#4650=CYLINDRICAL_SURFACE('',#20808,0.6);
#4651=CYLINDRICAL_SURFACE('',#20813,0.6);
#4652=CYLINDRICAL_SURFACE('',#20818,0.6);
#4653=CYLINDRICAL_SURFACE('',#20823,0.6);
#4654=CYLINDRICAL_SURFACE('',#20828,0.6);
#4655=CYLINDRICAL_SURFACE('',#20834,0.6);
#4656=CYLINDRICAL_SURFACE('',#20836,0.6);
#4657=CYLINDRICAL_SURFACE('',#20840,0.6);
#4658=CYLINDRICAL_SURFACE('',#20841,0.6);
#4659=CYLINDRICAL_SURFACE('',#20846,0.6);
#4660=CYLINDRICAL_SURFACE('',#20849,0.6);
#4661=CYLINDRICAL_SURFACE('',#20851,0.6);
#4662=CYLINDRICAL_SURFACE('',#20853,0.6);
#4663=CYLINDRICAL_SURFACE('',#20854,0.6);
#4664=CYLINDRICAL_SURFACE('',#20859,7.5888);
#4665=CYLINDRICAL_SURFACE('',#20861,0.6);
#4666=CYLINDRICAL_SURFACE('',#20864,0.6);
#4667=CYLINDRICAL_SURFACE('',#20865,1.632);
#4668=CYLINDRICAL_SURFACE('',#20869,0.6);
#4669=CYLINDRICAL_SURFACE('',#20875,0.6);
#4670=CYLINDRICAL_SURFACE('',#20878,2.856);
#5113=FACE_OUTER_BOUND('',#6279,.T.);
#5114=FACE_OUTER_BOUND('',#6280,.T.);
#5115=FACE_OUTER_BOUND('',#6281,.T.);
#5116=FACE_OUTER_BOUND('',#6282,.T.);
#5117=FACE_OUTER_BOUND('',#6283,.T.);
#5118=FACE_OUTER_BOUND('',#6284,.T.);
#5119=FACE_OUTER_BOUND('',#6285,.T.);
#5120=FACE_OUTER_BOUND('',#6286,.T.);
#5121=FACE_OUTER_BOUND('',#6287,.T.);
#5122=FACE_OUTER_BOUND('',#6288,.T.);
#5123=FACE_OUTER_BOUND('',#6289,.T.);
#5124=FACE_OUTER_BOUND('',#6290,.T.);
#5125=FACE_OUTER_BOUND('',#6291,.T.);
#5126=FACE_OUTER_BOUND('',#6292,.T.);
#5127=FACE_OUTER_BOUND('',#6293,.T.);
#5128=FACE_OUTER_BOUND('',#6294,.T.);
#5129=FACE_OUTER_BOUND('',#6295,.T.);
#5130=FACE_OUTER_BOUND('',#6296,.T.);
#5131=FACE_OUTER_BOUND('',#6297,.T.);
#5132=FACE_OUTER_BOUND('',#6298,.T.);
#5133=FACE_OUTER_BOUND('',#6299,.T.);
#5134=FACE_OUTER_BOUND('',#6300,.T.);
#5135=FACE_OUTER_BOUND('',#6301,.T.);
#5136=FACE_OUTER_BOUND('',#6302,.T.);
#5137=FACE_OUTER_BOUND('',#6303,.T.);
#5138=FACE_OUTER_BOUND('',#6304,.T.);
#5139=FACE_OUTER_BOUND('',#6305,.T.);
#5140=FACE_OUTER_BOUND('',#6306,.T.);
#5141=FACE_OUTER_BOUND('',#6307,.T.);
#5142=FACE_OUTER_BOUND('',#6308,.T.);
#5143=FACE_OUTER_BOUND('',#6309,.T.);
#5144=FACE_OUTER_BOUND('',#6310,.T.);
#5145=FACE_OUTER_BOUND('',#6311,.T.);
#5146=FACE_OUTER_BOUND('',#6312,.T.);
#5147=FACE_OUTER_BOUND('',#6313,.T.);
#5148=FACE_OUTER_BOUND('',#6314,.T.);
#5149=FACE_OUTER_BOUND('',#6315,.T.);
#5150=FACE_OUTER_BOUND('',#6323,.T.);
#5151=FACE_OUTER_BOUND('',#6324,.T.);
#5152=FACE_OUTER_BOUND('',#6325,.T.);
#5153=FACE_OUTER_BOUND('',#6326,.T.);
#5154=FACE_OUTER_BOUND('',#6327,.T.);
#5155=FACE_OUTER_BOUND('',#6328,.T.);
#5156=FACE_OUTER_BOUND('',#6329,.T.);
#5157=FACE_OUTER_BOUND('',#6330,.T.);
#5158=FACE_OUTER_BOUND('',#6331,.T.);
#5159=FACE_OUTER_BOUND('',#6332,.T.);
#5160=FACE_OUTER_BOUND('',#6333,.T.);
#5161=FACE_OUTER_BOUND('',#6334,.T.);
#5162=FACE_OUTER_BOUND('',#6335,.T.);
#5163=FACE_OUTER_BOUND('',#6336,.T.);
#5164=FACE_OUTER_BOUND('',#6337,.T.);
#5165=FACE_OUTER_BOUND('',#6338,.T.);
#5166=FACE_OUTER_BOUND('',#6339,.T.);
#5167=FACE_OUTER_BOUND('',#6340,.T.);
#5168=FACE_OUTER_BOUND('',#6341,.T.);
#5169=FACE_OUTER_BOUND('',#6342,.T.);
#5170=FACE_OUTER_BOUND('',#6343,.T.);
#5171=FACE_OUTER_BOUND('',#6344,.T.);
#5172=FACE_OUTER_BOUND('',#6345,.T.);
#5173=FACE_OUTER_BOUND('',#6346,.T.);
#5174=FACE_OUTER_BOUND('',#6347,.T.);
#5175=FACE_OUTER_BOUND('',#6348,.T.);
#5176=FACE_OUTER_BOUND('',#6349,.T.);
#5177=FACE_OUTER_BOUND('',#6350,.T.);
#5178=FACE_OUTER_BOUND('',#6351,.T.);
#5179=FACE_OUTER_BOUND('',#6352,.T.);
#5180=FACE_OUTER_BOUND('',#6353,.T.);
#5181=FACE_OUTER_BOUND('',#6354,.T.);
#5182=FACE_OUTER_BOUND('',#6355,.T.);
#5183=FACE_OUTER_BOUND('',#6356,.T.);
#5184=FACE_OUTER_BOUND('',#6357,.T.);
#5185=FACE_OUTER_BOUND('',#6358,.T.);
#5186=FACE_OUTER_BOUND('',#6359,.T.);
#5187=FACE_OUTER_BOUND('',#6360,.T.);
#5188=FACE_OUTER_BOUND('',#6361,.T.);
#5189=FACE_OUTER_BOUND('',#6362,.T.);
#5190=FACE_OUTER_BOUND('',#6363,.T.);
#5191=FACE_OUTER_BOUND('',#6364,.T.);
#5192=FACE_OUTER_BOUND('',#6365,.T.);
#5193=FACE_OUTER_BOUND('',#6366,.T.);
#5194=FACE_OUTER_BOUND('',#6367,.T.);
#5195=FACE_OUTER_BOUND('',#6368,.T.);
#5196=FACE_OUTER_BOUND('',#6369,.T.);
#5197=FACE_OUTER_BOUND('',#6370,.T.);
#5198=FACE_OUTER_BOUND('',#6371,.T.);
#5199=FACE_OUTER_BOUND('',#6372,.T.);
#5200=FACE_OUTER_BOUND('',#6373,.T.);
#5201=FACE_OUTER_BOUND('',#6374,.T.);
#5202=FACE_OUTER_BOUND('',#6375,.T.);
#5203=FACE_OUTER_BOUND('',#6376,.T.);
#5204=FACE_OUTER_BOUND('',#6377,.T.);
#5205=FACE_OUTER_BOUND('',#6378,.T.);
#5206=FACE_OUTER_BOUND('',#6379,.T.);
#5207=FACE_OUTER_BOUND('',#6380,.T.);
#5208=FACE_OUTER_BOUND('',#6381,.T.);
#5209=FACE_OUTER_BOUND('',#6382,.T.);
#5210=FACE_OUTER_BOUND('',#6383,.T.);
#5211=FACE_OUTER_BOUND('',#6384,.T.);
#5212=FACE_OUTER_BOUND('',#6385,.T.);
#5213=FACE_OUTER_BOUND('',#6386,.T.);
#5214=FACE_OUTER_BOUND('',#6387,.T.);
#5215=FACE_OUTER_BOUND('',#6388,.T.);
#5216=FACE_OUTER_BOUND('',#6389,.T.);
#5217=FACE_OUTER_BOUND('',#6390,.T.);
#5218=FACE_OUTER_BOUND('',#6391,.T.);
#5219=FACE_OUTER_BOUND('',#6392,.T.);
#5220=FACE_OUTER_BOUND('',#6393,.T.);
#5221=FACE_OUTER_BOUND('',#6394,.T.);
#5222=FACE_OUTER_BOUND('',#6395,.T.);
#5223=FACE_OUTER_BOUND('',#6396,.T.);
#5224=FACE_OUTER_BOUND('',#6397,.T.);
#5225=FACE_OUTER_BOUND('',#6398,.T.);
#5226=FACE_OUTER_BOUND('',#6399,.T.);
#5227=FACE_OUTER_BOUND('',#6400,.T.);
#5228=FACE_OUTER_BOUND('',#6401,.T.);
#5229=FACE_OUTER_BOUND('',#6402,.T.);
#5230=FACE_OUTER_BOUND('',#6403,.T.);
#5231=FACE_OUTER_BOUND('',#6404,.T.);
#5232=FACE_OUTER_BOUND('',#6405,.T.);
#5233=FACE_OUTER_BOUND('',#6406,.T.);
#5234=FACE_OUTER_BOUND('',#6407,.T.);
#5235=FACE_OUTER_BOUND('',#6408,.T.);
#5236=FACE_OUTER_BOUND('',#6409,.T.);
#5237=FACE_OUTER_BOUND('',#6410,.T.);
#5238=FACE_OUTER_BOUND('',#6411,.T.);
#5239=FACE_OUTER_BOUND('',#6412,.T.);
#5240=FACE_OUTER_BOUND('',#6413,.T.);
#5241=FACE_OUTER_BOUND('',#6414,.T.);
#5242=FACE_OUTER_BOUND('',#6415,.T.);
#5243=FACE_OUTER_BOUND('',#6416,.T.);
#5244=FACE_OUTER_BOUND('',#6417,.T.);
#5245=FACE_OUTER_BOUND('',#6418,.T.);
#5246=FACE_OUTER_BOUND('',#6419,.T.);
#5247=FACE_OUTER_BOUND('',#6420,.T.);
#5248=FACE_OUTER_BOUND('',#6421,.T.);
#5249=FACE_OUTER_BOUND('',#6422,.T.);
#5250=FACE_OUTER_BOUND('',#6423,.T.);
#5251=FACE_OUTER_BOUND('',#6431,.T.);
#5252=FACE_OUTER_BOUND('',#6432,.T.);
#5253=FACE_OUTER_BOUND('',#6433,.T.);
#5254=FACE_OUTER_BOUND('',#6434,.T.);
#5255=FACE_OUTER_BOUND('',#6435,.T.);
#5256=FACE_OUTER_BOUND('',#6436,.T.);
#5257=FACE_OUTER_BOUND('',#6437,.T.);
#5258=FACE_OUTER_BOUND('',#6438,.T.);
#5259=FACE_OUTER_BOUND('',#6439,.T.);
#5260=FACE_OUTER_BOUND('',#6440,.T.);
#5261=FACE_OUTER_BOUND('',#6441,.T.);
#5262=FACE_OUTER_BOUND('',#6442,.T.);
#5263=FACE_OUTER_BOUND('',#6443,.T.);
#5264=FACE_OUTER_BOUND('',#6444,.T.);
#5265=FACE_OUTER_BOUND('',#6445,.T.);
#5266=FACE_OUTER_BOUND('',#6446,.T.);
#5267=FACE_OUTER_BOUND('',#6447,.T.);
#5268=FACE_OUTER_BOUND('',#6448,.T.);
#5269=FACE_OUTER_BOUND('',#6449,.T.);
#5270=FACE_OUTER_BOUND('',#6450,.T.);
#5271=FACE_OUTER_BOUND('',#6451,.T.);
#5272=FACE_OUTER_BOUND('',#6452,.T.);
#5273=FACE_OUTER_BOUND('',#6453,.T.);
#5274=FACE_OUTER_BOUND('',#6454,.T.);
#5275=FACE_OUTER_BOUND('',#6455,.T.);
#5276=FACE_OUTER_BOUND('',#6456,.T.);
#5277=FACE_OUTER_BOUND('',#6457,.T.);
#5278=FACE_OUTER_BOUND('',#6458,.T.);
#5279=FACE_OUTER_BOUND('',#6459,.T.);
#5280=FACE_OUTER_BOUND('',#6460,.T.);
#5281=FACE_OUTER_BOUND('',#6461,.T.);
#5282=FACE_OUTER_BOUND('',#6462,.T.);
#5283=FACE_OUTER_BOUND('',#6463,.T.);
#5284=FACE_OUTER_BOUND('',#6464,.T.);
#5285=FACE_OUTER_BOUND('',#6465,.T.);
#5286=FACE_OUTER_BOUND('',#6466,.T.);
#5287=FACE_OUTER_BOUND('',#6467,.T.);
#5288=FACE_OUTER_BOUND('',#6468,.T.);
#5289=FACE_OUTER_BOUND('',#6469,.T.);
#5290=FACE_OUTER_BOUND('',#6470,.T.);
#5291=FACE_OUTER_BOUND('',#6471,.T.);
#5292=FACE_OUTER_BOUND('',#6472,.T.);
#5293=FACE_OUTER_BOUND('',#6473,.T.);
#5294=FACE_OUTER_BOUND('',#6474,.T.);
#5295=FACE_OUTER_BOUND('',#6475,.T.);
#5296=FACE_OUTER_BOUND('',#6476,.T.);
#5297=FACE_OUTER_BOUND('',#6477,.T.);
#5298=FACE_OUTER_BOUND('',#6478,.T.);
#5299=FACE_OUTER_BOUND('',#6479,.T.);
#5300=FACE_OUTER_BOUND('',#6480,.T.);
#5301=FACE_OUTER_BOUND('',#6481,.T.);
#5302=FACE_OUTER_BOUND('',#6482,.T.);
#5303=FACE_OUTER_BOUND('',#6483,.T.);
#5304=FACE_OUTER_BOUND('',#6484,.T.);
#5305=FACE_OUTER_BOUND('',#6485,.T.);
#5306=FACE_OUTER_BOUND('',#6486,.T.);
#5307=FACE_OUTER_BOUND('',#6487,.T.);
#5308=FACE_OUTER_BOUND('',#6488,.T.);
#5309=FACE_OUTER_BOUND('',#6489,.T.);
#5310=FACE_OUTER_BOUND('',#6490,.T.);
#5311=FACE_OUTER_BOUND('',#6491,.T.);
#5312=FACE_OUTER_BOUND('',#6492,.T.);
#5313=FACE_OUTER_BOUND('',#6493,.T.);
#5314=FACE_OUTER_BOUND('',#6494,.T.);
#5315=FACE_OUTER_BOUND('',#6495,.T.);
#5316=FACE_OUTER_BOUND('',#6496,.T.);
#5317=FACE_OUTER_BOUND('',#6497,.T.);
#5318=FACE_OUTER_BOUND('',#6498,.T.);
#5319=FACE_OUTER_BOUND('',#6499,.T.);
#5320=FACE_OUTER_BOUND('',#6500,.T.);
#5321=FACE_OUTER_BOUND('',#6501,.T.);
#5322=FACE_OUTER_BOUND('',#6502,.T.);
#5323=FACE_OUTER_BOUND('',#6503,.T.);
#5324=FACE_OUTER_BOUND('',#6504,.T.);
#5325=FACE_OUTER_BOUND('',#6505,.T.);
#5326=FACE_OUTER_BOUND('',#6506,.T.);
#5327=FACE_OUTER_BOUND('',#6507,.T.);
#5328=FACE_OUTER_BOUND('',#6508,.T.);
#5329=FACE_OUTER_BOUND('',#6509,.T.);
#5330=FACE_OUTER_BOUND('',#6510,.T.);
#5331=FACE_OUTER_BOUND('',#6511,.T.);
#5332=FACE_OUTER_BOUND('',#6512,.T.);
#5333=FACE_OUTER_BOUND('',#6513,.T.);
#5334=FACE_OUTER_BOUND('',#6514,.T.);
#5335=FACE_OUTER_BOUND('',#6515,.T.);
#5336=FACE_OUTER_BOUND('',#6516,.T.);
#5337=FACE_OUTER_BOUND('',#6517,.T.);
#5338=FACE_OUTER_BOUND('',#6518,.T.);
#5339=FACE_OUTER_BOUND('',#6519,.T.);
#5340=FACE_OUTER_BOUND('',#6520,.T.);
#5341=FACE_OUTER_BOUND('',#6521,.T.);
#5342=FACE_OUTER_BOUND('',#6522,.T.);
#5343=FACE_OUTER_BOUND('',#6523,.T.);
#5344=FACE_OUTER_BOUND('',#6524,.T.);
#5345=FACE_OUTER_BOUND('',#6525,.T.);
#5346=FACE_OUTER_BOUND('',#6526,.T.);
#5347=FACE_OUTER_BOUND('',#6527,.T.);
#5348=FACE_OUTER_BOUND('',#6528,.T.);
#5349=FACE_OUTER_BOUND('',#6529,.T.);
#5350=FACE_OUTER_BOUND('',#6530,.T.);
#5351=FACE_OUTER_BOUND('',#6531,.T.);
#5352=FACE_OUTER_BOUND('',#6532,.T.);
#5353=FACE_OUTER_BOUND('',#6533,.T.);
#5354=FACE_OUTER_BOUND('',#6534,.T.);
#5355=FACE_OUTER_BOUND('',#6535,.T.);
#5356=FACE_OUTER_BOUND('',#6536,.T.);
#5357=FACE_OUTER_BOUND('',#6537,.T.);
#5358=FACE_OUTER_BOUND('',#6538,.T.);
#6279=EDGE_LOOP('',(#13539,#13540,#13541,#13542,#13543,#13544));
#6280=EDGE_LOOP('',(#13545,#13546,#13547,#13548,#13549,#13550));
#6281=EDGE_LOOP('',(#13551,#13552,#13553,#13554,#13555,#13556));
#6282=EDGE_LOOP('',(#13557,#13558,#13559,#13560));
#6283=EDGE_LOOP('',(#13561,#13562,#13563));
#6284=EDGE_LOOP('',(#13564,#13565,#13566));
#6285=EDGE_LOOP('',(#13567,#13568,#13569,#13570));
#6286=EDGE_LOOP('',(#13571,#13572,#13573,#13574));
#6287=EDGE_LOOP('',(#13575,#13576,#13577,#13578));
#6288=EDGE_LOOP('',(#13579,#13580,#13581,#13582));
#6289=EDGE_LOOP('',(#13583,#13584,#13585));
#6290=EDGE_LOOP('',(#13586,#13587,#13588));
#6291=EDGE_LOOP('',(#13589,#13590,#13591,#13592));
#6292=EDGE_LOOP('',(#13593,#13594,#13595,#13596));
#6293=EDGE_LOOP('',(#13597,#13598,#13599,#13600));
#6294=EDGE_LOOP('',(#13601,#13602,#13603));
#6295=EDGE_LOOP('',(#13604,#13605,#13606));
#6296=EDGE_LOOP('',(#13607,#13608,#13609,#13610));
#6297=EDGE_LOOP('',(#13611,#13612,#13613,#13614));
#6298=EDGE_LOOP('',(#13615,#13616,#13617,#13618));
#6299=EDGE_LOOP('',(#13619,#13620,#13621));
#6300=EDGE_LOOP('',(#13622,#13623,#13624));
#6301=EDGE_LOOP('',(#13625,#13626,#13627,#13628));
#6302=EDGE_LOOP('',(#13629,#13630,#13631,#13632));
#6303=EDGE_LOOP('',(#13633,#13634,#13635,#13636));
#6304=EDGE_LOOP('',(#13637,#13638,#13639));
#6305=EDGE_LOOP('',(#13640,#13641,#13642));
#6306=EDGE_LOOP('',(#13643,#13644,#13645,#13646));
#6307=EDGE_LOOP('',(#13647,#13648,#13649,#13650));
#6308=EDGE_LOOP('',(#13651,#13652,#13653,#13654));
#6309=EDGE_LOOP('',(#13655,#13656,#13657,#13658));
#6310=EDGE_LOOP('',(#13659,#13660,#13661));
#6311=EDGE_LOOP('',(#13662,#13663,#13664));
#6312=EDGE_LOOP('',(#13665,#13666,#13667,#13668));
#6313=EDGE_LOOP('',(#13669,#13670,#13671,#13672));
#6314=EDGE_LOOP('',(#13673,#13674,#13675,#13676,#13677));
#6315=EDGE_LOOP('',(#13678,#13679,#13680,#13681,#13682,#13683,#13684,#13685,
#13686,#13687,#13688,#13689,#13690,#13691,#13692,#13693,#13694,#13695,#13696,
#13697,#13698,#13699,#13700,#13701));
#6316=EDGE_LOOP('',(#13702));
#6317=EDGE_LOOP('',(#13703,#13704,#13705,#13706));
#6318=EDGE_LOOP('',(#13707,#13708,#13709,#13710,#13711,#13712,#13713,#13714));
#6319=EDGE_LOOP('',(#13715));
#6320=EDGE_LOOP('',(#13716,#13717,#13718,#13719,#13720,#13721,#13722,#13723));
#6321=EDGE_LOOP('',(#13724));
#6322=EDGE_LOOP('',(#13725));
#6323=EDGE_LOOP('',(#13726,#13727,#13728,#13729,#13730,#13731));
#6324=EDGE_LOOP('',(#13732,#13733,#13734,#13735,#13736));
#6325=EDGE_LOOP('',(#13737,#13738,#13739,#13740,#13741,#13742));
#6326=EDGE_LOOP('',(#13743,#13744,#13745,#13746,#13747));
#6327=EDGE_LOOP('',(#13748,#13749,#13750,#13751));
#6328=EDGE_LOOP('',(#13752,#13753,#13754,#13755));
#6329=EDGE_LOOP('',(#13756,#13757,#13758,#13759));
#6330=EDGE_LOOP('',(#13760,#13761,#13762,#13763));
#6331=EDGE_LOOP('',(#13764,#13765,#13766,#13767));
#6332=EDGE_LOOP('',(#13768,#13769,#13770,#13771));
#6333=EDGE_LOOP('',(#13772,#13773,#13774,#13775));
#6334=EDGE_LOOP('',(#13776,#13777,#13778,#13779));
#6335=EDGE_LOOP('',(#13780,#13781,#13782));
#6336=EDGE_LOOP('',(#13783,#13784,#13785,#13786));
#6337=EDGE_LOOP('',(#13787,#13788,#13789));
#6338=EDGE_LOOP('',(#13790,#13791,#13792,#13793));
#6339=EDGE_LOOP('',(#13794,#13795,#13796,#13797));
#6340=EDGE_LOOP('',(#13798,#13799,#13800,#13801));
#6341=EDGE_LOOP('',(#13802,#13803,#13804,#13805));
#6342=EDGE_LOOP('',(#13806,#13807,#13808));
#6343=EDGE_LOOP('',(#13809,#13810,#13811,#13812));
#6344=EDGE_LOOP('',(#13813,#13814,#13815));
#6345=EDGE_LOOP('',(#13816,#13817,#13818));
#6346=EDGE_LOOP('',(#13819,#13820,#13821,#13822));
#6347=EDGE_LOOP('',(#13823,#13824,#13825));
#6348=EDGE_LOOP('',(#13826,#13827,#13828,#13829));
#6349=EDGE_LOOP('',(#13830,#13831,#13832));
#6350=EDGE_LOOP('',(#13833,#13834,#13835,#13836));
#6351=EDGE_LOOP('',(#13837,#13838,#13839,#13840));
#6352=EDGE_LOOP('',(#13841,#13842,#13843));
#6353=EDGE_LOOP('',(#13844,#13845,#13846,#13847));
#6354=EDGE_LOOP('',(#13848,#13849,#13850));
#6355=EDGE_LOOP('',(#13851,#13852,#13853,#13854));
#6356=EDGE_LOOP('',(#13855,#13856,#13857));
#6357=EDGE_LOOP('',(#13858,#13859,#13860,#13861));
#6358=EDGE_LOOP('',(#13862,#13863,#13864));
#6359=EDGE_LOOP('',(#13865,#13866,#13867,#13868));
#6360=EDGE_LOOP('',(#13869,#13870,#13871,#13872));
#6361=EDGE_LOOP('',(#13873,#13874,#13875,#13876));
#6362=EDGE_LOOP('',(#13877,#13878,#13879,#13880));
#6363=EDGE_LOOP('',(#13881,#13882,#13883,#13884));
#6364=EDGE_LOOP('',(#13885,#13886,#13887));
#6365=EDGE_LOOP('',(#13888,#13889,#13890));
#6366=EDGE_LOOP('',(#13891,#13892,#13893,#13894));
#6367=EDGE_LOOP('',(#13895,#13896,#13897,#13898));
#6368=EDGE_LOOP('',(#13899,#13900,#13901));
#6369=EDGE_LOOP('',(#13902,#13903,#13904,#13905));
#6370=EDGE_LOOP('',(#13906,#13907,#13908,#13909));
#6371=EDGE_LOOP('',(#13910,#13911,#13912,#13913));
#6372=EDGE_LOOP('',(#13914,#13915,#13916,#13917));
#6373=EDGE_LOOP('',(#13918,#13919,#13920,#13921));
#6374=EDGE_LOOP('',(#13922,#13923,#13924));
#6375=EDGE_LOOP('',(#13925,#13926,#13927,#13928));
#6376=EDGE_LOOP('',(#13929,#13930,#13931));
#6377=EDGE_LOOP('',(#13932,#13933,#13934,#13935));
#6378=EDGE_LOOP('',(#13936,#13937,#13938,#13939));
#6379=EDGE_LOOP('',(#13940,#13941,#13942,#13943));
#6380=EDGE_LOOP('',(#13944,#13945,#13946,#13947));
#6381=EDGE_LOOP('',(#13948,#13949,#13950,#13951));
#6382=EDGE_LOOP('',(#13952,#13953,#13954,#13955));
#6383=EDGE_LOOP('',(#13956,#13957,#13958,#13959,#13960));
#6384=EDGE_LOOP('',(#13961,#13962,#13963,#13964,#13965,#13966));
#6385=EDGE_LOOP('',(#13967,#13968,#13969));
#6386=EDGE_LOOP('',(#13970,#13971,#13972,#13973));
#6387=EDGE_LOOP('',(#13974,#13975,#13976));
#6388=EDGE_LOOP('',(#13977,#13978,#13979,#13980));
#6389=EDGE_LOOP('',(#13981,#13982,#13983));
#6390=EDGE_LOOP('',(#13984,#13985,#13986,#13987));
#6391=EDGE_LOOP('',(#13988,#13989,#13990));
#6392=EDGE_LOOP('',(#13991,#13992,#13993,#13994));
#6393=EDGE_LOOP('',(#13995,#13996,#13997,#13998));
#6394=EDGE_LOOP('',(#13999,#14000,#14001,#14002));
#6395=EDGE_LOOP('',(#14003,#14004,#14005));
#6396=EDGE_LOOP('',(#14006,#14007,#14008,#14009));
#6397=EDGE_LOOP('',(#14010,#14011,#14012,#14013));
#6398=EDGE_LOOP('',(#14014,#14015,#14016,#14017));
#6399=EDGE_LOOP('',(#14018,#14019,#14020));
#6400=EDGE_LOOP('',(#14021,#14022,#14023,#14024));
#6401=EDGE_LOOP('',(#14025,#14026,#14027));
#6402=EDGE_LOOP('',(#14028,#14029,#14030,#14031));
#6403=EDGE_LOOP('',(#14032,#14033,#14034));
#6404=EDGE_LOOP('',(#14035,#14036,#14037,#14038));
#6405=EDGE_LOOP('',(#14039,#14040,#14041));
#6406=EDGE_LOOP('',(#14042,#14043,#14044,#14045));
#6407=EDGE_LOOP('',(#14046,#14047,#14048));
#6408=EDGE_LOOP('',(#14049,#14050,#14051,#14052));
#6409=EDGE_LOOP('',(#14053,#14054,#14055));
#6410=EDGE_LOOP('',(#14056,#14057,#14058,#14059));
#6411=EDGE_LOOP('',(#14060,#14061,#14062,#14063));
#6412=EDGE_LOOP('',(#14064,#14065,#14066,#14067));
#6413=EDGE_LOOP('',(#14068,#14069,#14070,#14071));
#6414=EDGE_LOOP('',(#14072,#14073,#14074,#14075));
#6415=EDGE_LOOP('',(#14076,#14077,#14078,#14079));
#6416=EDGE_LOOP('',(#14080,#14081,#14082,#14083));
#6417=EDGE_LOOP('',(#14084,#14085,#14086,#14087));
#6418=EDGE_LOOP('',(#14088,#14089,#14090,#14091));
#6419=EDGE_LOOP('',(#14092,#14093,#14094,#14095));
#6420=EDGE_LOOP('',(#14096,#14097,#14098,#14099));
#6421=EDGE_LOOP('',(#14100,#14101,#14102,#14103));
#6422=EDGE_LOOP('',(#14104,#14105,#14106,#14107,#14108));
#6423=EDGE_LOOP('',(#14109,#14110,#14111,#14112,#14113,#14114,#14115,#14116,
#14117,#14118,#14119,#14120,#14121,#14122,#14123,#14124,#14125,#14126,#14127,
#14128,#14129,#14130,#14131,#14132));
#6424=EDGE_LOOP('',(#14133,#14134,#14135,#14136,#14137,#14138,#14139,#14140));
#6425=EDGE_LOOP('',(#14141,#14142,#14143,#14144));
#6426=EDGE_LOOP('',(#14145));
#6427=EDGE_LOOP('',(#14146,#14147,#14148,#14149,#14150,#14151,#14152,#14153));
#6428=EDGE_LOOP('',(#14154));
#6429=EDGE_LOOP('',(#14155));
#6430=EDGE_LOOP('',(#14156));
#6431=EDGE_LOOP('',(#14157,#14158,#14159));
#6432=EDGE_LOOP('',(#14160,#14161,#14162,#14163));
#6433=EDGE_LOOP('',(#14164,#14165,#14166,#14167));
#6434=EDGE_LOOP('',(#14168,#14169,#14170,#14171));
#6435=EDGE_LOOP('',(#14172,#14173,#14174));
#6436=EDGE_LOOP('',(#14175,#14176,#14177));
#6437=EDGE_LOOP('',(#14178,#14179,#14180,#14181));
#6438=EDGE_LOOP('',(#14182,#14183,#14184,#14185));
#6439=EDGE_LOOP('',(#14186,#14187,#14188,#14189));
#6440=EDGE_LOOP('',(#14190,#14191,#14192,#14193));
#6441=EDGE_LOOP('',(#14194,#14195,#14196,#14197));
#6442=EDGE_LOOP('',(#14198,#14199,#14200));
#6443=EDGE_LOOP('',(#14201,#14202,#14203,#14204));
#6444=EDGE_LOOP('',(#14205,#14206,#14207,#14208));
#6445=EDGE_LOOP('',(#14209,#14210,#14211,#14212));
#6446=EDGE_LOOP('',(#14213,#14214,#14215,#14216));
#6447=EDGE_LOOP('',(#14217,#14218,#14219,#14220));
#6448=EDGE_LOOP('',(#14221,#14222,#14223));
#6449=EDGE_LOOP('',(#14224,#14225,#14226));
#6450=EDGE_LOOP('',(#14227,#14228,#14229,#14230));
#6451=EDGE_LOOP('',(#14231,#14232,#14233));
#6452=EDGE_LOOP('',(#14234,#14235,#14236,#14237));
#6453=EDGE_LOOP('',(#14238,#14239,#14240,#14241));
#6454=EDGE_LOOP('',(#14242,#14243,#14244));
#6455=EDGE_LOOP('',(#14245,#14246,#14247));
#6456=EDGE_LOOP('',(#14248,#14249,#14250,#14251));
#6457=EDGE_LOOP('',(#14252,#14253,#14254));
#6458=EDGE_LOOP('',(#14255,#14256,#14257,#14258));
#6459=EDGE_LOOP('',(#14259,#14260,#14261,#14262));
#6460=EDGE_LOOP('',(#14263,#14264,#14265));
#6461=EDGE_LOOP('',(#14266,#14267,#14268,#14269));
#6462=EDGE_LOOP('',(#14270,#14271,#14272,#14273));
#6463=EDGE_LOOP('',(#14274,#14275,#14276));
#6464=EDGE_LOOP('',(#14277,#14278,#14279,#14280));
#6465=EDGE_LOOP('',(#14281,#14282,#14283));
#6466=EDGE_LOOP('',(#14284,#14285,#14286,#14287));
#6467=EDGE_LOOP('',(#14288,#14289,#14290,#14291));
#6468=EDGE_LOOP('',(#14292,#14293,#14294,#14295));
#6469=EDGE_LOOP('',(#14296,#14297,#14298));
#6470=EDGE_LOOP('',(#14299,#14300,#14301,#14302));
#6471=EDGE_LOOP('',(#14303,#14304,#14305,#14306));
#6472=EDGE_LOOP('',(#14307,#14308,#14309,#14310));
#6473=EDGE_LOOP('',(#14311,#14312,#14313));
#6474=EDGE_LOOP('',(#14314,#14315,#14316,#14317));
#6475=EDGE_LOOP('',(#14318,#14319,#14320,#14321));
#6476=EDGE_LOOP('',(#14322,#14323,#14324,#14325));
#6477=EDGE_LOOP('',(#14326,#14327,#14328));
#6478=EDGE_LOOP('',(#14329,#14330,#14331,#14332));
#6479=EDGE_LOOP('',(#14333,#14334,#14335,#14336));
#6480=EDGE_LOOP('',(#14337,#14338,#14339,#14340));
#6481=EDGE_LOOP('',(#14341,#14342,#14343));
#6482=EDGE_LOOP('',(#14344,#14345,#14346,#14347));
#6483=EDGE_LOOP('',(#14348,#14349,#14350));
#6484=EDGE_LOOP('',(#14351,#14352,#14353,#14354));
#6485=EDGE_LOOP('',(#14355,#14356,#14357));
#6486=EDGE_LOOP('',(#14358,#14359,#14360,#14361));
#6487=EDGE_LOOP('',(#14362,#14363,#14364,#14365));
#6488=EDGE_LOOP('',(#14366,#14367,#14368,#14369));
#6489=EDGE_LOOP('',(#14370,#14371,#14372,#14373));
#6490=EDGE_LOOP('',(#14374,#14375,#14376,#14377));
#6491=EDGE_LOOP('',(#14378,#14379,#14380));
#6492=EDGE_LOOP('',(#14381,#14382,#14383,#14384));
#6493=EDGE_LOOP('',(#14385,#14386,#14387));
#6494=EDGE_LOOP('',(#14388,#14389,#14390,#14391));
#6495=EDGE_LOOP('',(#14392,#14393,#14394));
#6496=EDGE_LOOP('',(#14395,#14396,#14397,#14398));
#6497=EDGE_LOOP('',(#14399,#14400,#14401));
#6498=EDGE_LOOP('',(#14402,#14403,#14404,#14405));
#6499=EDGE_LOOP('',(#14406,#14407,#14408));
#6500=EDGE_LOOP('',(#14409,#14410,#14411));
#6501=EDGE_LOOP('',(#14412,#14413,#14414,#14415));
#6502=EDGE_LOOP('',(#14416,#14417,#14418,#14419));
#6503=EDGE_LOOP('',(#14420,#14421,#14422,#14423));
#6504=EDGE_LOOP('',(#14424,#14425,#14426,#14427));
#6505=EDGE_LOOP('',(#14428,#14429,#14430,#14431));
#6506=EDGE_LOOP('',(#14432,#14433,#14434,#14435));
#6507=EDGE_LOOP('',(#14436,#14437,#14438,#14439));
#6508=EDGE_LOOP('',(#14440,#14441,#14442,#14443));
#6509=EDGE_LOOP('',(#14444,#14445,#14446,#14447));
#6510=EDGE_LOOP('',(#14448,#14449,#14450,#14451));
#6511=EDGE_LOOP('',(#14452,#14453,#14454,#14455));
#6512=EDGE_LOOP('',(#14456,#14457,#14458,#14459));
#6513=EDGE_LOOP('',(#14460,#14461,#14462,#14463));
#6514=EDGE_LOOP('',(#14464,#14465,#14466,#14467));
#6515=EDGE_LOOP('',(#14468,#14469,#14470,#14471));
#6516=EDGE_LOOP('',(#14472,#14473,#14474,#14475));
#6517=EDGE_LOOP('',(#14476,#14477,#14478,#14479));
#6518=EDGE_LOOP('',(#14480,#14481,#14482,#14483));
#6519=EDGE_LOOP('',(#14484,#14485,#14486,#14487));
#6520=EDGE_LOOP('',(#14488,#14489,#14490,#14491));
#6521=EDGE_LOOP('',(#14492,#14493,#14494,#14495));
#6522=EDGE_LOOP('',(#14496,#14497,#14498,#14499));
#6523=EDGE_LOOP('',(#14500,#14501,#14502,#14503));
#6524=EDGE_LOOP('',(#14504,#14505,#14506,#14507));
#6525=EDGE_LOOP('',(#14508,#14509,#14510,#14511));
#6526=EDGE_LOOP('',(#14512,#14513,#14514,#14515));
#6527=EDGE_LOOP('',(#14516,#14517,#14518,#14519,#14520));
#6528=EDGE_LOOP('',(#14521,#14522,#14523,#14524));
#6529=EDGE_LOOP('',(#14525,#14526,#14527,#14528));
#6530=EDGE_LOOP('',(#14529,#14530,#14531,#14532));
#6531=EDGE_LOOP('',(#14533,#14534,#14535,#14536));
#6532=EDGE_LOOP('',(#14537,#14538,#14539,#14540));
#6533=EDGE_LOOP('',(#14541,#14542,#14543,#14544,#14545));
#6534=EDGE_LOOP('',(#14546,#14547,#14548,#14549,#14550));
#6535=EDGE_LOOP('',(#14551,#14552,#14553,#14554,#14555,#14556));
#6536=EDGE_LOOP('',(#14557,#14558,#14559,#14560,#14561,#14562));
#6537=EDGE_LOOP('',(#14563,#14564,#14565,#14566));
#6538=EDGE_LOOP('',(#14567,#14568,#14569,#14570));
#8279=VERTEX_POINT('',#59067);
#8280=VERTEX_POINT('',#59068);
#8281=VERTEX_POINT('',#59070);
#8282=VERTEX_POINT('',#59072);
#8283=VERTEX_POINT('',#59077);
#8284=VERTEX_POINT('',#59078);
#8285=VERTEX_POINT('',#59083);
#8286=VERTEX_POINT('',#59085);
#8287=VERTEX_POINT('',#59089);
#8288=VERTEX_POINT('',#59090);
#8289=VERTEX_POINT('',#59092);
#8290=VERTEX_POINT('',#59094);
#8291=VERTEX_POINT('',#59098);
#8292=VERTEX_POINT('',#59102);
#8293=VERTEX_POINT('',#59106);
#8294=VERTEX_POINT('',#59108);
#8295=VERTEX_POINT('',#59112);
#8296=VERTEX_POINT('',#59114);
#8297=VERTEX_POINT('',#59118);
#8298=VERTEX_POINT('',#59122);
#8299=VERTEX_POINT('',#59124);
#8300=VERTEX_POINT('',#59126);
#8301=VERTEX_POINT('',#59130);
#8302=VERTEX_POINT('',#59136);
#8303=VERTEX_POINT('',#59138);
#8304=VERTEX_POINT('',#59144);
#8305=VERTEX_POINT('',#59145);
#8306=VERTEX_POINT('',#59148);
#8307=VERTEX_POINT('',#59154);
#8308=VERTEX_POINT('',#59158);
#8309=VERTEX_POINT('',#59160);
#8310=VERTEX_POINT('',#59166);
#8311=VERTEX_POINT('',#59168);
#8312=VERTEX_POINT('',#59170);
#8313=VERTEX_POINT('',#59174);
#8314=VERTEX_POINT('',#59180);
#8315=VERTEX_POINT('',#59182);
#8316=VERTEX_POINT('',#59188);
#8317=VERTEX_POINT('',#59189);
#8318=VERTEX_POINT('',#59191);
#8319=VERTEX_POINT('',#59193);
#8320=VERTEX_POINT('',#59197);
#8321=VERTEX_POINT('',#59201);
#8322=VERTEX_POINT('',#59205);
#8323=VERTEX_POINT('',#59207);
#8324=VERTEX_POINT('',#59211);
#8325=VERTEX_POINT('',#59213);
#8326=VERTEX_POINT('',#59217);
#8327=VERTEX_POINT('',#59221);
#8328=VERTEX_POINT('',#59222);
#8329=VERTEX_POINT('',#59225);
#8330=VERTEX_POINT('',#59231);
#8331=VERTEX_POINT('',#59235);
#8332=VERTEX_POINT('',#59237);
#8333=VERTEX_POINT('',#59243);
#8334=VERTEX_POINT('',#59245);
#8335=VERTEX_POINT('',#59247);
#8336=VERTEX_POINT('',#59251);
#8337=VERTEX_POINT('',#59252);
#8338=VERTEX_POINT('',#59254);
#8339=VERTEX_POINT('',#59256);
#8340=VERTEX_POINT('',#59258);
#8341=VERTEX_POINT('',#59260);
#8342=VERTEX_POINT('',#59262);
#8343=VERTEX_POINT('',#59264);
#8344=VERTEX_POINT('',#59266);
#8345=VERTEX_POINT('',#59268);
#8346=VERTEX_POINT('',#59270);
#8347=VERTEX_POINT('',#59272);
#8348=VERTEX_POINT('',#59274);
#8349=VERTEX_POINT('',#59276);
#8350=VERTEX_POINT('',#59278);
#8351=VERTEX_POINT('',#59280);
#8352=VERTEX_POINT('',#59282);
#8353=VERTEX_POINT('',#59284);
#8354=VERTEX_POINT('',#59286);
#8355=VERTEX_POINT('',#59288);
#8356=VERTEX_POINT('',#59290);
#8357=VERTEX_POINT('',#59292);
#8358=VERTEX_POINT('',#59294);
#8359=VERTEX_POINT('',#59296);
#8360=VERTEX_POINT('',#59299);
#8361=VERTEX_POINT('',#59301);
#8362=VERTEX_POINT('',#59302);
#8363=VERTEX_POINT('',#59304);
#8364=VERTEX_POINT('',#59306);
#8365=VERTEX_POINT('',#59309);
#8366=VERTEX_POINT('',#59311);
#8367=VERTEX_POINT('',#59313);
#8368=VERTEX_POINT('',#59315);
#8369=VERTEX_POINT('',#59317);
#8370=VERTEX_POINT('',#59319);
#8371=VERTEX_POINT('',#59323);
#8372=VERTEX_POINT('',#59325);
#8373=VERTEX_POINT('',#59326);
#8374=VERTEX_POINT('',#59328);
#8375=VERTEX_POINT('',#59334);
#8376=VERTEX_POINT('',#59337);
#8377=VERTEX_POINT('',#59340);
#8378=VERTEX_POINT('',#59342);
#8379=VERTEX_POINT('',#59346);
#8380=VERTEX_POINT('',#59348);
#8381=VERTEX_POINT('',#59352);
#8382=VERTEX_POINT('',#59354);
#8383=VERTEX_POINT('',#59360);
#8384=VERTEX_POINT('',#59362);
#8385=VERTEX_POINT('',#59366);
#8386=VERTEX_POINT('',#59370);
#8387=VERTEX_POINT('',#59376);
#8388=VERTEX_POINT('',#59378);
#8389=VERTEX_POINT('',#59382);
#8390=VERTEX_POINT('',#59386);
#8391=VERTEX_POINT('',#59392);
#8392=VERTEX_POINT('',#59397);
#8393=VERTEX_POINT('',#59403);
#8394=VERTEX_POINT('',#59407);
#8395=VERTEX_POINT('',#59411);
#8396=VERTEX_POINT('',#59413);
#8397=VERTEX_POINT('',#59417);
#8398=VERTEX_POINT('',#59421);
#8399=VERTEX_POINT('',#59425);
#8400=VERTEX_POINT('',#59426);
#8401=VERTEX_POINT('',#59431);
#8402=VERTEX_POINT('',#59433);
#8403=VERTEX_POINT('',#59439);
#8404=VERTEX_POINT('',#59440);
#8405=VERTEX_POINT('',#59447);
#8406=VERTEX_POINT('',#59448);
#8407=VERTEX_POINT('',#59455);
#8408=VERTEX_POINT('',#59459);
#8409=VERTEX_POINT('',#59463);
#8410=VERTEX_POINT('',#59464);
#8411=VERTEX_POINT('',#59469);
#8412=VERTEX_POINT('',#59473);
#8413=VERTEX_POINT('',#59474);
#8414=VERTEX_POINT('',#59479);
#8415=VERTEX_POINT('',#59483);
#8416=VERTEX_POINT('',#59484);
#8417=VERTEX_POINT('',#59489);
#8418=VERTEX_POINT('',#59499);
#8419=VERTEX_POINT('',#59501);
#8420=VERTEX_POINT('',#59507);
#8421=VERTEX_POINT('',#59509);
#8422=VERTEX_POINT('',#59513);
#8423=VERTEX_POINT('',#59514);
#8424=VERTEX_POINT('',#59516);
#8425=VERTEX_POINT('',#59523);
#8426=VERTEX_POINT('',#59527);
#8427=VERTEX_POINT('',#59531);
#8428=VERTEX_POINT('',#59535);
#8429=VERTEX_POINT('',#59543);
#8430=VERTEX_POINT('',#59550);
#8431=VERTEX_POINT('',#59552);
#8432=VERTEX_POINT('',#59556);
#8433=VERTEX_POINT('',#59567);
#8434=VERTEX_POINT('',#59571);
#8435=VERTEX_POINT('',#59573);
#8436=VERTEX_POINT('',#59577);
#8437=VERTEX_POINT('',#59579);
#8438=VERTEX_POINT('',#59583);
#8439=VERTEX_POINT('',#59584);
#8440=VERTEX_POINT('',#59591);
#8441=VERTEX_POINT('',#59592);
#8442=VERTEX_POINT('',#59599);
#8443=VERTEX_POINT('',#59600);
#8444=VERTEX_POINT('',#59607);
#8445=VERTEX_POINT('',#59608);
#8446=VERTEX_POINT('',#59615);
#8447=VERTEX_POINT('',#59619);
#8448=VERTEX_POINT('',#59623);
#8449=VERTEX_POINT('',#59624);
#8450=VERTEX_POINT('',#59633);
#8451=VERTEX_POINT('',#59634);
#8452=VERTEX_POINT('',#59639);
#8453=VERTEX_POINT('',#59643);
#8454=VERTEX_POINT('',#59644);
#8455=VERTEX_POINT('',#59649);
#8456=VERTEX_POINT('',#59653);
#8457=VERTEX_POINT('',#59654);
#8458=VERTEX_POINT('',#59659);
#8459=VERTEX_POINT('',#59663);
#8460=VERTEX_POINT('',#59664);
#8461=VERTEX_POINT('',#59669);
#8462=VERTEX_POINT('',#59673);
#8463=VERTEX_POINT('',#59674);
#8464=VERTEX_POINT('',#59679);
#8465=VERTEX_POINT('',#59683);
#8466=VERTEX_POINT('',#59700);
#8467=VERTEX_POINT('',#59702);
#8468=VERTEX_POINT('',#59708);
#8469=VERTEX_POINT('',#59714);
#8470=VERTEX_POINT('',#59718);
#8471=VERTEX_POINT('',#59720);
#8472=VERTEX_POINT('',#59726);
#8473=VERTEX_POINT('',#59730);
#8474=VERTEX_POINT('',#59732);
#8475=VERTEX_POINT('',#59734);
#8476=VERTEX_POINT('',#59736);
#8477=VERTEX_POINT('',#59738);
#8478=VERTEX_POINT('',#59740);
#8479=VERTEX_POINT('',#59742);
#8480=VERTEX_POINT('',#59744);
#8481=VERTEX_POINT('',#59746);
#8482=VERTEX_POINT('',#59748);
#8483=VERTEX_POINT('',#59750);
#8484=VERTEX_POINT('',#59752);
#8485=VERTEX_POINT('',#59758);
#8486=VERTEX_POINT('',#59760);
#8487=VERTEX_POINT('',#59762);
#8488=VERTEX_POINT('',#59764);
#8489=VERTEX_POINT('',#59767);
#8490=VERTEX_POINT('',#59768);
#8491=VERTEX_POINT('',#59770);
#8492=VERTEX_POINT('',#59772);
#8493=VERTEX_POINT('',#59775);
#8494=VERTEX_POINT('',#59778);
#8495=VERTEX_POINT('',#59780);
#8496=VERTEX_POINT('',#59785);
#8497=VERTEX_POINT('',#59803);
#8498=VERTEX_POINT('',#59805);
#8499=VERTEX_POINT('',#59817);
#8500=VERTEX_POINT('',#59821);
#8501=VERTEX_POINT('',#59822);
#8502=VERTEX_POINT('',#59829);
#8503=VERTEX_POINT('',#59831);
#8504=VERTEX_POINT('',#59837);
#8505=VERTEX_POINT('',#59838);
#8506=VERTEX_POINT('',#59846);
#8507=VERTEX_POINT('',#59847);
#8508=VERTEX_POINT('',#59860);
#8509=VERTEX_POINT('',#59866);
#8510=VERTEX_POINT('',#59870);
#8511=VERTEX_POINT('',#59874);
#8512=VERTEX_POINT('',#59878);
#8513=VERTEX_POINT('',#59879);
#8514=VERTEX_POINT('',#59890);
#8515=VERTEX_POINT('',#59899);
#8516=VERTEX_POINT('',#59903);
#8517=VERTEX_POINT('',#59904);
#8518=VERTEX_POINT('',#59909);
#8519=VERTEX_POINT('',#59915);
#8520=VERTEX_POINT('',#59919);
#8521=VERTEX_POINT('',#59920);
#8522=VERTEX_POINT('',#59927);
#8523=VERTEX_POINT('',#59931);
#8524=VERTEX_POINT('',#59935);
#8525=VERTEX_POINT('',#59936);
#8526=VERTEX_POINT('',#59943);
#8527=VERTEX_POINT('',#59944);
#8528=VERTEX_POINT('',#59951);
#8529=VERTEX_POINT('',#59952);
#8530=VERTEX_POINT('',#59961);
#8531=VERTEX_POINT('',#59962);
#8532=VERTEX_POINT('',#59970);
#8533=VERTEX_POINT('',#59971);
#8534=VERTEX_POINT('',#59979);
#8535=VERTEX_POINT('',#59980);
#8536=VERTEX_POINT('',#59988);
#8537=VERTEX_POINT('',#59989);
#8538=VERTEX_POINT('',#59997);
#8539=VERTEX_POINT('',#59998);
#8540=VERTEX_POINT('',#60006);
#8541=VERTEX_POINT('',#60015);
#8542=VERTEX_POINT('',#60019);
#8543=VERTEX_POINT('',#60028);
#8544=VERTEX_POINT('',#60034);
#8545=VERTEX_POINT('',#60050);
#8546=VERTEX_POINT('',#60073);
#8547=VERTEX_POINT('',#60085);
#8548=VERTEX_POINT('',#60086);
#8549=VERTEX_POINT('',#60091);
#8550=VERTEX_POINT('',#60092);
#10244=EDGE_CURVE('',#8279,#8280,#250,.T.);
#10245=EDGE_CURVE('',#8280,#8281,#251,.T.);
#10246=EDGE_CURVE('',#8281,#8282,#252,.T.);
#10247=EDGE_CURVE('',#8282,#8281,#253,.T.);
#10248=EDGE_CURVE('',#8280,#8279,#254,.T.);
#10249=EDGE_CURVE('',#8283,#8284,#255,.T.);
#10250=EDGE_CURVE('',#8284,#8283,#256,.T.);
#10251=EDGE_CURVE('',#8284,#8282,#2070,.T.);
#10252=EDGE_CURVE('',#8279,#8285,#2071,.T.);
#10253=EDGE_CURVE('',#8286,#8285,#257,.T.);
#10254=EDGE_CURVE('',#8285,#8286,#258,.T.);
#10255=EDGE_CURVE('',#8287,#8288,#259,.T.);
#10256=EDGE_CURVE('',#8288,#8289,#2072,.T.);
#10257=EDGE_CURVE('',#8289,#8290,#260,.T.);
#10258=EDGE_CURVE('',#8290,#8287,#2073,.T.);
#10259=EDGE_CURVE('',#8289,#8291,#261,.T.);
#10260=EDGE_CURVE('',#8291,#8290,#262,.T.);
#10261=EDGE_CURVE('',#8287,#8292,#263,.T.);
#10262=EDGE_CURVE('',#8292,#8288,#264,.T.);
#10263=EDGE_CURVE('',#8291,#8293,#2074,.T.);
#10264=EDGE_CURVE('',#8294,#8293,#265,.T.);
#10265=EDGE_CURVE('',#8294,#8290,#2075,.T.);
#10266=EDGE_CURVE('',#8289,#8295,#266,.T.);
#10267=EDGE_CURVE('',#8295,#8296,#267,.F.);
#10268=EDGE_CURVE('',#8296,#8291,#268,.T.);
#10269=EDGE_CURVE('',#8297,#8288,#269,.T.);
#10270=EDGE_CURVE('',#8295,#8297,#2076,.T.);
#10271=EDGE_CURVE('',#8294,#8298,#270,.T.);
#10272=EDGE_CURVE('',#8298,#8299,#2077,.T.);
#10273=EDGE_CURVE('',#8299,#8300,#271,.T.);
#10274=EDGE_CURVE('',#8300,#8294,#2078,.T.);
#10275=EDGE_CURVE('',#8299,#8301,#272,.T.);
#10276=EDGE_CURVE('',#8301,#8300,#273,.T.);
#10277=EDGE_CURVE('',#8293,#8298,#274,.T.);
#10278=EDGE_CURVE('',#8293,#8302,#275,.T.);
#10279=EDGE_CURVE('',#8303,#8302,#276,.T.);
#10280=EDGE_CURVE('',#8303,#8298,#277,.T.);
#10281=EDGE_CURVE('',#8287,#8300,#2079,.T.);
#10282=EDGE_CURVE('',#8304,#8305,#278,.T.);
#10283=EDGE_CURVE('',#8305,#8303,#2080,.T.);
#10284=EDGE_CURVE('',#8303,#8306,#279,.T.);
#10285=EDGE_CURVE('',#8306,#8304,#2081,.T.);
#10286=EDGE_CURVE('',#8302,#8306,#280,.T.);
#10287=EDGE_CURVE('',#8304,#8307,#281,.T.);
#10288=EDGE_CURVE('',#8307,#8305,#282,.T.);
#10289=EDGE_CURVE('',#8302,#8308,#2082,.T.);
#10290=EDGE_CURVE('',#8309,#8308,#283,.T.);
#10291=EDGE_CURVE('',#8309,#8306,#2083,.T.);
#10292=EDGE_CURVE('',#8299,#8305,#284,.T.);
#10293=EDGE_CURVE('',#8309,#8310,#285,.T.);
#10294=EDGE_CURVE('',#8310,#8311,#2084,.T.);
#10295=EDGE_CURVE('',#8311,#8312,#286,.T.);
#10296=EDGE_CURVE('',#8312,#8309,#2085,.T.);
#10297=EDGE_CURVE('',#8311,#8313,#287,.T.);
#10298=EDGE_CURVE('',#8313,#8312,#288,.T.);
#10299=EDGE_CURVE('',#8308,#8310,#289,.T.);
#10300=EDGE_CURVE('',#8308,#8314,#290,.T.);
#10301=EDGE_CURVE('',#8314,#8315,#291,.T.);
#10302=EDGE_CURVE('',#8315,#8310,#292,.T.);
#10303=EDGE_CURVE('',#8304,#8312,#2086,.T.);
#10304=EDGE_CURVE('',#8316,#8317,#293,.T.);
#10305=EDGE_CURVE('',#8317,#8318,#2087,.T.);
#10306=EDGE_CURVE('',#8318,#8319,#294,.T.);
#10307=EDGE_CURVE('',#8319,#8316,#2088,.T.);
#10308=EDGE_CURVE('',#8318,#8320,#295,.T.);
#10309=EDGE_CURVE('',#8320,#8319,#296,.T.);
#10310=EDGE_CURVE('',#8316,#8321,#297,.T.);
#10311=EDGE_CURVE('',#8321,#8317,#298,.T.);
#10312=EDGE_CURVE('',#8321,#8322,#299,.T.);
#10313=EDGE_CURVE('',#8323,#8322,#300,.T.);
#10314=EDGE_CURVE('',#8323,#8317,#301,.T.);
#10315=EDGE_CURVE('',#8316,#8324,#2089,.T.);
#10316=EDGE_CURVE('',#8325,#8324,#302,.T.);
#10317=EDGE_CURVE('',#8325,#8321,#2090,.T.);
#10318=EDGE_CURVE('',#8326,#8319,#2091,.T.);
#10319=EDGE_CURVE('',#8324,#8326,#2092,.T.);
#10320=EDGE_CURVE('',#8327,#8328,#303,.T.);
#10321=EDGE_CURVE('',#8328,#8323,#2093,.T.);
#10322=EDGE_CURVE('',#8323,#8329,#304,.T.);
#10323=EDGE_CURVE('',#8329,#8327,#2094,.T.);
#10324=EDGE_CURVE('',#8322,#8329,#305,.T.);
#10325=EDGE_CURVE('',#8327,#8330,#306,.T.);
#10326=EDGE_CURVE('',#8330,#8328,#307,.T.);
#10327=EDGE_CURVE('',#8322,#8331,#2095,.T.);
#10328=EDGE_CURVE('',#8332,#8331,#308,.T.);
#10329=EDGE_CURVE('',#8332,#8329,#2096,.T.);
#10330=EDGE_CURVE('',#8318,#8328,#309,.T.);
#10331=EDGE_CURVE('',#8333,#8333,#310,.T.);
#10332=EDGE_CURVE('',#8333,#8334,#311,.T.);
#10333=EDGE_CURVE('',#8334,#8335,#312,.T.);
#10334=EDGE_CURVE('',#8335,#8334,#313,.T.);
#10335=EDGE_CURVE('',#8336,#8337,#2097,.T.);
#10336=EDGE_CURVE('',#8338,#8336,#2098,.T.);
#10337=EDGE_CURVE('',#8339,#8338,#2099,.T.);
#10338=EDGE_CURVE('',#8340,#8339,#2100,.T.);
#10339=EDGE_CURVE('',#8341,#8340,#2101,.T.);
#10340=EDGE_CURVE('',#8342,#8341,#2102,.T.);
#10341=EDGE_CURVE('',#8343,#8342,#2103,.T.);
#10342=EDGE_CURVE('',#8344,#8343,#2104,.T.);
#10343=EDGE_CURVE('',#8345,#8344,#2105,.T.);
#10344=EDGE_CURVE('',#8346,#8345,#2106,.T.);
#10345=EDGE_CURVE('',#8347,#8346,#2107,.T.);
#10346=EDGE_CURVE('',#8348,#8347,#2108,.T.);
#10347=EDGE_CURVE('',#8349,#8348,#2109,.T.);
#10348=EDGE_CURVE('',#8350,#8349,#2110,.T.);
#10349=EDGE_CURVE('',#8351,#8350,#2111,.T.);
#10350=EDGE_CURVE('',#8352,#8351,#2112,.T.);
#10351=EDGE_CURVE('',#8353,#8352,#2113,.T.);
#10352=EDGE_CURVE('',#8354,#8353,#2114,.T.);
#10353=EDGE_CURVE('',#8355,#8354,#2115,.T.);
#10354=EDGE_CURVE('',#8356,#8355,#2116,.T.);
#10355=EDGE_CURVE('',#8357,#8356,#2117,.T.);
#10356=EDGE_CURVE('',#8358,#8357,#2118,.T.);
#10357=EDGE_CURVE('',#8359,#8358,#314,.T.);
#10358=EDGE_CURVE('',#8337,#8359,#2119,.T.);
#10359=EDGE_CURVE('',#8360,#8360,#315,.T.);
#10360=EDGE_CURVE('',#8361,#8362,#2120,.T.);
#10361=EDGE_CURVE('',#8363,#8361,#316,.T.);
#10362=EDGE_CURVE('',#8364,#8363,#2121,.T.);
#10363=EDGE_CURVE('',#8362,#8364,#317,.T.);
#10364=EDGE_CURVE('',#8365,#8330,#2122,.T.);
#10365=EDGE_CURVE('',#8366,#8365,#318,.T.);
#10366=EDGE_CURVE('',#8367,#8366,#2123,.T.);
#10367=EDGE_CURVE('',#8368,#8367,#319,.T.);
#10368=EDGE_CURVE('',#8369,#8368,#2124,.T.);
#10369=EDGE_CURVE('',#8370,#8369,#320,.T.);
#10370=EDGE_CURVE('',#8320,#8370,#2125,.T.);
#10371=EDGE_CURVE('',#8330,#8320,#321,.T.);
#10372=EDGE_CURVE('',#8371,#8371,#322,.T.);
#10373=EDGE_CURVE('',#8372,#8373,#323,.T.);
#10374=EDGE_CURVE('',#8374,#8372,#2126,.T.);
#10375=EDGE_CURVE('',#8292,#8374,#324,.T.);
#10376=EDGE_CURVE('',#8301,#8292,#2127,.T.);
#10377=EDGE_CURVE('',#8307,#8301,#325,.T.);
#10378=EDGE_CURVE('',#8313,#8307,#2128,.T.);
#10379=EDGE_CURVE('',#8375,#8313,#326,.T.);
#10380=EDGE_CURVE('',#8373,#8375,#2129,.T.);
#10381=EDGE_CURVE('',#8376,#8376,#327,.T.);
#10382=EDGE_CURVE('',#8335,#8377,#2130,.T.);
#10383=EDGE_CURVE('',#8378,#8377,#328,.T.);
#10384=EDGE_CURVE('',#8377,#8378,#329,.T.);
#10385=EDGE_CURVE('',#8360,#8379,#330,.T.);
#10386=EDGE_CURVE('',#8379,#8380,#331,.T.);
#10387=EDGE_CURVE('',#8380,#8379,#332,.T.);
#10388=EDGE_CURVE('',#8380,#8381,#2131,.T.);
#10389=EDGE_CURVE('',#8382,#8381,#333,.T.);
#10390=EDGE_CURVE('',#8381,#8382,#334,.T.);
#10391=EDGE_CURVE('',#8376,#8283,#335,.T.);
#10392=EDGE_CURVE('',#8362,#8383,#336,.T.);
#10393=EDGE_CURVE('',#8383,#8384,#2132,.T.);
#10394=EDGE_CURVE('',#8384,#8361,#337,.T.);
#10395=EDGE_CURVE('',#8385,#8363,#338,.T.);
#10396=EDGE_CURVE('',#8384,#8385,#339,.T.);
#10397=EDGE_CURVE('',#8386,#8364,#340,.T.);
#10398=EDGE_CURVE('',#8385,#8386,#2133,.T.);
#10399=EDGE_CURVE('',#8386,#8383,#341,.T.);
#10400=EDGE_CURVE('',#8384,#8387,#2134,.T.);
#10401=EDGE_CURVE('',#8388,#8387,#342,.T.);
#10402=EDGE_CURVE('',#8385,#8388,#2135,.T.);
#10403=EDGE_CURVE('',#8383,#8389,#2136,.T.);
#10404=EDGE_CURVE('',#8387,#8389,#2137,.T.);
#10405=EDGE_CURVE('',#8327,#8390,#2138,.T.);
#10406=EDGE_CURVE('',#8390,#8365,#343,.T.);
#10407=EDGE_CURVE('',#8326,#8370,#344,.T.);
#10408=EDGE_CURVE('',#8370,#8391,#345,.T.);
#10409=EDGE_CURVE('',#8391,#8326,#346,.T.);
#10410=EDGE_CURVE('',#8390,#8392,#347,.T.);
#10411=EDGE_CURVE('',#8392,#8365,#348,.T.);
#10412=EDGE_CURVE('',#8390,#8332,#2139,.T.);
#10413=EDGE_CURVE('',#8391,#8393,#2140,.T.);
#10414=EDGE_CURVE('',#8393,#8324,#349,.T.);
#10415=EDGE_CURVE('',#8369,#8394,#350,.F.);
#10416=EDGE_CURVE('',#8394,#8391,#351,.T.);
#10417=EDGE_CURVE('',#8395,#8336,#1813,.F.);
#10418=EDGE_CURVE('',#8337,#8396,#352,.T.);
#10419=EDGE_CURVE('',#8396,#8395,#2141,.T.);
#10420=EDGE_CURVE('',#8337,#8397,#353,.T.);
#10421=EDGE_CURVE('',#8397,#8396,#354,.T.);
#10422=EDGE_CURVE('',#8359,#8398,#355,.T.);
#10423=EDGE_CURVE('',#8398,#8397,#2142,.T.);
#10424=EDGE_CURVE('',#8399,#8400,#356,.F.);
#10425=EDGE_CURVE('',#8348,#8399,#357,.F.);
#10426=EDGE_CURVE('',#8400,#8348,#358,.F.);
#10427=EDGE_CURVE('',#8349,#8401,#359,.T.);
#10428=EDGE_CURVE('',#8401,#8402,#360,.T.);
#10429=EDGE_CURVE('',#8402,#8349,#361,.T.);
#10430=EDGE_CURVE('',#8399,#8401,#2143,.T.);
#10431=EDGE_CURVE('',#8403,#8404,#362,.F.);
#10432=EDGE_CURVE('',#8347,#8403,#363,.F.);
#10433=EDGE_CURVE('',#8404,#8347,#364,.F.);
#10434=EDGE_CURVE('',#8403,#8400,#2144,.T.);
#10435=EDGE_CURVE('',#8405,#8406,#365,.F.);
#10436=EDGE_CURVE('',#8346,#8405,#366,.F.);
#10437=EDGE_CURVE('',#8406,#8346,#367,.F.);
#10438=EDGE_CURVE('',#8405,#8404,#2145,.T.);
#10439=EDGE_CURVE('',#8345,#8407,#368,.T.);
#10440=EDGE_CURVE('',#8407,#8406,#2146,.T.);
#10441=EDGE_CURVE('',#8345,#8408,#369,.T.);
#10442=EDGE_CURVE('',#8408,#8407,#370,.T.);
#10443=EDGE_CURVE('',#8409,#8410,#371,.T.);
#10444=EDGE_CURVE('',#8410,#8405,#2147,.T.);
#10445=EDGE_CURVE('',#8406,#8409,#2148,.T.);
#10446=EDGE_CURVE('',#8409,#8411,#372,.T.);
#10447=EDGE_CURVE('',#8411,#8410,#373,.T.);
#10448=EDGE_CURVE('',#8412,#8413,#374,.T.);
#10449=EDGE_CURVE('',#8413,#8403,#2149,.T.);
#10450=EDGE_CURVE('',#8404,#8412,#2150,.T.);
#10451=EDGE_CURVE('',#8412,#8414,#375,.T.);
#10452=EDGE_CURVE('',#8414,#8413,#376,.T.);
#10453=EDGE_CURVE('',#8415,#8416,#377,.T.);
#10454=EDGE_CURVE('',#8416,#8399,#2151,.T.);
#10455=EDGE_CURVE('',#8400,#8415,#2152,.T.);
#10456=EDGE_CURVE('',#8415,#8417,#378,.T.);
#10457=EDGE_CURVE('',#8417,#8416,#379,.T.);
#10458=EDGE_CURVE('',#8415,#8413,#2153,.T.);
#10459=EDGE_CURVE('',#8412,#8410,#2154,.T.);
#10460=EDGE_CURVE('',#8411,#8414,#2155,.T.);
#10461=EDGE_CURVE('',#8409,#8418,#2156,.T.);
#10462=EDGE_CURVE('',#8419,#8418,#380,.T.);
#10463=EDGE_CURVE('',#8419,#8411,#2157,.T.);
#10464=EDGE_CURVE('',#8418,#8407,#2158,.T.);
#10465=EDGE_CURVE('',#8420,#8373,#381,.F.);
#10466=EDGE_CURVE('',#8421,#8420,#382,.F.);
#10467=EDGE_CURVE('',#8373,#8421,#383,.F.);
#10468=EDGE_CURVE('',#8422,#8423,#384,.T.);
#10469=EDGE_CURVE('',#8423,#8424,#385,.T.);
#10470=EDGE_CURVE('',#8424,#8422,#386,.T.);
#10471=EDGE_CURVE('',#8422,#8421,#2159,.T.);
#10472=EDGE_CURVE('',#8420,#8423,#2160,.T.);
#10473=EDGE_CURVE('',#8425,#8372,#387,.T.);
#10474=EDGE_CURVE('',#8421,#8425,#388,.T.);
#10475=EDGE_CURVE('',#8425,#8426,#389,.T.);
#10476=EDGE_CURVE('',#8426,#8372,#390,.T.);
#10477=EDGE_CURVE('',#8375,#8427,#391,.T.);
#10478=EDGE_CURVE('',#8427,#8420,#2161,.T.);
#10479=EDGE_CURVE('',#8311,#8428,#392,.T.);
#10480=EDGE_CURVE('',#8428,#8375,#393,.T.);
#10481=EDGE_CURVE('',#8297,#8374,#394,.T.);
#10482=EDGE_CURVE('',#8374,#8429,#395,.T.);
#10483=EDGE_CURVE('',#8429,#8297,#396,.T.);
#10484=EDGE_CURVE('',#8428,#8427,#397,.T.);
#10485=EDGE_CURVE('',#8424,#8430,#398,.T.);
#10486=EDGE_CURVE('',#8431,#8430,#399,.T.);
#10487=EDGE_CURVE('',#8431,#8422,#400,.T.);
#10488=EDGE_CURVE('',#8423,#8432,#2162,.T.);
#10489=EDGE_CURVE('',#8314,#8432,#401,.T.);
#10490=EDGE_CURVE('',#8314,#8424,#2163,.T.);
#10491=EDGE_CURVE('',#8432,#8427,#2164,.T.);
#10492=EDGE_CURVE('',#8428,#8315,#2165,.T.);
#10493=EDGE_CURVE('',#8315,#8432,#402,.T.);
#10494=EDGE_CURVE('',#8429,#8433,#2166,.T.);
#10495=EDGE_CURVE('',#8433,#8295,#403,.F.);
#10496=EDGE_CURVE('',#8371,#8434,#404,.T.);
#10497=EDGE_CURVE('',#8434,#8435,#405,.T.);
#10498=EDGE_CURVE('',#8435,#8434,#406,.T.);
#10499=EDGE_CURVE('',#8435,#8436,#2167,.T.);
#10500=EDGE_CURVE('',#8437,#8436,#407,.T.);
#10501=EDGE_CURVE('',#8436,#8437,#408,.T.);
#10502=EDGE_CURVE('',#8438,#8439,#409,.F.);
#10503=EDGE_CURVE('',#8344,#8438,#410,.F.);
#10504=EDGE_CURVE('',#8439,#8344,#411,.F.);
#10505=EDGE_CURVE('',#8438,#8408,#2168,.T.);
#10506=EDGE_CURVE('',#8440,#8441,#412,.F.);
#10507=EDGE_CURVE('',#8343,#8440,#413,.F.);
#10508=EDGE_CURVE('',#8441,#8343,#414,.F.);
#10509=EDGE_CURVE('',#8440,#8439,#2169,.T.);
#10510=EDGE_CURVE('',#8442,#8443,#415,.F.);
#10511=EDGE_CURVE('',#8342,#8442,#416,.F.);
#10512=EDGE_CURVE('',#8443,#8342,#417,.F.);
#10513=EDGE_CURVE('',#8442,#8441,#2170,.T.);
#10514=EDGE_CURVE('',#8444,#8445,#418,.F.);
#10515=EDGE_CURVE('',#8341,#8444,#419,.F.);
#10516=EDGE_CURVE('',#8445,#8341,#420,.F.);
#10517=EDGE_CURVE('',#8444,#8443,#2171,.T.);
#10518=EDGE_CURVE('',#8446,#8445,#2172,.T.);
#10519=EDGE_CURVE('',#8340,#8446,#1814,.T.);
#10520=EDGE_CURVE('',#8339,#8447,#1815,.T.);
#10521=EDGE_CURVE('',#8447,#8446,#2173,.T.);
#10522=EDGE_CURVE('',#8448,#8449,#421,.F.);
#10523=EDGE_CURVE('',#8338,#8448,#422,.F.);
#10524=EDGE_CURVE('',#8449,#8338,#423,.F.);
#10525=EDGE_CURVE('',#8448,#8447,#2174,.T.);
#10526=EDGE_CURVE('',#8395,#8449,#2175,.T.);
#10527=EDGE_CURVE('',#8450,#8451,#424,.T.);
#10528=EDGE_CURVE('',#8451,#8448,#2176,.T.);
#10529=EDGE_CURVE('',#8449,#8450,#2177,.T.);
#10530=EDGE_CURVE('',#8450,#8452,#425,.T.);
#10531=EDGE_CURVE('',#8452,#8451,#426,.T.);
#10532=EDGE_CURVE('',#8453,#8454,#427,.T.);
#10533=EDGE_CURVE('',#8454,#8444,#2178,.T.);
#10534=EDGE_CURVE('',#8445,#8453,#2179,.T.);
#10535=EDGE_CURVE('',#8453,#8455,#428,.T.);
#10536=EDGE_CURVE('',#8455,#8454,#429,.T.);
#10537=EDGE_CURVE('',#8456,#8457,#430,.T.);
#10538=EDGE_CURVE('',#8457,#8442,#2180,.T.);
#10539=EDGE_CURVE('',#8443,#8456,#2181,.T.);
#10540=EDGE_CURVE('',#8456,#8458,#431,.T.);
#10541=EDGE_CURVE('',#8458,#8457,#432,.T.);
#10542=EDGE_CURVE('',#8459,#8460,#433,.T.);
#10543=EDGE_CURVE('',#8460,#8440,#2182,.T.);
#10544=EDGE_CURVE('',#8441,#8459,#2183,.T.);
#10545=EDGE_CURVE('',#8459,#8461,#434,.T.);
#10546=EDGE_CURVE('',#8461,#8460,#435,.T.);
#10547=EDGE_CURVE('',#8462,#8463,#436,.T.);
#10548=EDGE_CURVE('',#8463,#8438,#2184,.T.);
#10549=EDGE_CURVE('',#8439,#8462,#2185,.T.);
#10550=EDGE_CURVE('',#8462,#8464,#437,.T.);
#10551=EDGE_CURVE('',#8464,#8463,#438,.T.);
#10552=EDGE_CURVE('',#8408,#8465,#2186,.T.);
#10553=EDGE_CURVE('',#8465,#8418,#439,.T.);
#10554=EDGE_CURVE('',#8465,#8419,#440,.T.);
#10555=EDGE_CURVE('',#8459,#8457,#2187,.T.);
#10556=EDGE_CURVE('',#8461,#8464,#2188,.T.);
#10557=EDGE_CURVE('',#8462,#8460,#2189,.T.);
#10558=EDGE_CURVE('',#8458,#8461,#2190,.T.);
#10559=EDGE_CURVE('',#8456,#8454,#2191,.T.);
#10560=EDGE_CURVE('',#8455,#8458,#2192,.T.);
#10561=EDGE_CURVE('',#8453,#8466,#2193,.T.);
#10562=EDGE_CURVE('',#8467,#8466,#1816,.T.);
#10563=EDGE_CURVE('',#8467,#8455,#2194,.T.);
#10564=EDGE_CURVE('',#8446,#8466,#2195,.T.);
#10565=EDGE_CURVE('',#8447,#8468,#2196,.T.);
#10566=EDGE_CURVE('',#8466,#8468,#2197,.T.);
#10567=EDGE_CURVE('',#8468,#8451,#2198,.T.);
#10568=EDGE_CURVE('',#8452,#8469,#2199,.T.);
#10569=EDGE_CURVE('',#8469,#8468,#1817,.T.);
#10570=EDGE_CURVE('',#8450,#8470,#2200,.T.);
#10571=EDGE_CURVE('',#8470,#8471,#1818,.F.);
#10572=EDGE_CURVE('',#8471,#8452,#2201,.T.);
#10573=EDGE_CURVE('',#8395,#8470,#2202,.T.);
#10574=EDGE_CURVE('',#8472,#8472,#441,.T.);
#10575=EDGE_CURVE('',#8472,#8437,#442,.T.);
#10576=EDGE_CURVE('',#8473,#8471,#2203,.T.);
#10577=EDGE_CURVE('',#8474,#8473,#2204,.T.);
#10578=EDGE_CURVE('',#8475,#8474,#443,.T.);
#10579=EDGE_CURVE('',#8476,#8475,#2205,.T.);
#10580=EDGE_CURVE('',#8477,#8476,#2206,.T.);
#10581=EDGE_CURVE('',#8478,#8477,#2207,.T.);
#10582=EDGE_CURVE('',#8479,#8478,#2208,.T.);
#10583=EDGE_CURVE('',#8480,#8479,#2209,.T.);
#10584=EDGE_CURVE('',#8481,#8480,#2210,.T.);
#10585=EDGE_CURVE('',#8482,#8481,#2211,.T.);
#10586=EDGE_CURVE('',#8483,#8482,#2212,.T.);
#10587=EDGE_CURVE('',#8484,#8483,#2213,.T.);
#10588=EDGE_CURVE('',#8417,#8484,#2214,.T.);
#10589=EDGE_CURVE('',#8414,#8417,#2215,.T.);
#10590=EDGE_CURVE('',#8464,#8419,#2216,.T.);
#10591=EDGE_CURVE('',#8469,#8467,#2217,.T.);
#10592=EDGE_CURVE('',#8485,#8325,#444,.T.);
#10593=EDGE_CURVE('',#8486,#8485,#2218,.T.);
#10594=EDGE_CURVE('',#8487,#8486,#445,.T.);
#10595=EDGE_CURVE('',#8488,#8487,#2219,.T.);
#10596=EDGE_CURVE('',#8331,#8488,#446,.T.);
#10597=EDGE_CURVE('',#8489,#8490,#2220,.T.);
#10598=EDGE_CURVE('',#8491,#8489,#447,.T.);
#10599=EDGE_CURVE('',#8492,#8491,#2221,.T.);
#10600=EDGE_CURVE('',#8490,#8492,#448,.T.);
#10601=EDGE_CURVE('',#8493,#8493,#449,.T.);
#10602=EDGE_CURVE('',#8430,#8296,#2222,.T.);
#10603=EDGE_CURVE('',#8494,#8494,#450,.T.);
#10604=EDGE_CURVE('',#8495,#8495,#451,.T.);
#10605=EDGE_CURVE('',#8296,#8433,#452,.F.);
#10606=EDGE_CURVE('',#8496,#8430,#453,.T.);
#10607=EDGE_CURVE('',#8433,#8496,#2223,.T.);
#10608=EDGE_CURVE('',#8426,#8429,#2224,.T.);
#10609=EDGE_CURVE('',#8425,#8431,#2225,.T.);
#10610=EDGE_CURVE('',#8431,#8496,#454,.T.);
#10611=EDGE_CURVE('',#8496,#8426,#2226,.T.);
#10612=EDGE_CURVE('',#8465,#8463,#2227,.T.);
#10613=EDGE_CURVE('',#8497,#8484,#455,.T.);
#10614=EDGE_CURVE('',#8484,#8498,#456,.T.);
#10615=EDGE_CURVE('',#8498,#8497,#457,.T.);
#10616=EDGE_CURVE('',#8497,#8416,#2228,.T.);
#10617=EDGE_CURVE('',#8401,#8497,#2229,.T.);
#10618=EDGE_CURVE('',#8498,#8402,#2230,.T.);
#10619=EDGE_CURVE('',#8394,#8499,#458,.F.);
#10620=EDGE_CURVE('',#8499,#8369,#459,.F.);
#10621=EDGE_CURVE('',#8500,#8501,#460,.F.);
#10622=EDGE_CURVE('',#8368,#8500,#461,.F.);
#10623=EDGE_CURVE('',#8501,#8368,#462,.F.);
#10624=EDGE_CURVE('',#8500,#8499,#2231,.T.);
#10625=EDGE_CURVE('',#8502,#8367,#463,.T.);
#10626=EDGE_CURVE('',#8367,#8503,#464,.T.);
#10627=EDGE_CURVE('',#8503,#8502,#465,.T.);
#10628=EDGE_CURVE('',#8502,#8501,#466,.T.);
#10629=EDGE_CURVE('',#8504,#8505,#467,.T.);
#10630=EDGE_CURVE('',#8505,#8500,#2232,.T.);
#10631=EDGE_CURVE('',#8501,#8504,#2233,.T.);
#10632=EDGE_CURVE('',#8504,#8486,#468,.T.);
#10633=EDGE_CURVE('',#8486,#8505,#469,.T.);
#10634=EDGE_CURVE('',#8506,#8507,#470,.T.);
#10635=EDGE_CURVE('',#8507,#8485,#471,.T.);
#10636=EDGE_CURVE('',#8485,#8506,#472,.T.);
#10637=EDGE_CURVE('',#8506,#8394,#2234,.T.);
#10638=EDGE_CURVE('',#8499,#8507,#2235,.T.);
#10639=EDGE_CURVE('',#8393,#8325,#473,.T.);
#10640=EDGE_CURVE('',#8393,#8506,#474,.T.);
#10641=EDGE_CURVE('',#8508,#8332,#475,.T.);
#10642=EDGE_CURVE('',#8331,#8508,#476,.T.);
#10643=EDGE_CURVE('',#8508,#8392,#2236,.T.);
#10644=EDGE_CURVE('',#8392,#8509,#477,.T.);
#10645=EDGE_CURVE('',#8509,#8366,#478,.T.);
#10646=EDGE_CURVE('',#8509,#8510,#479,.T.);
#10647=EDGE_CURVE('',#8510,#8366,#480,.T.);
#10648=EDGE_CURVE('',#8511,#8488,#481,.T.);
#10649=EDGE_CURVE('',#8511,#8508,#482,.T.);
#10650=EDGE_CURVE('',#8512,#8513,#483,.T.);
#10651=EDGE_CURVE('',#8513,#8487,#484,.T.);
#10652=EDGE_CURVE('',#8487,#8512,#485,.T.);
#10653=EDGE_CURVE('',#8503,#8513,#2237,.T.);
#10654=EDGE_CURVE('',#8512,#8502,#2238,.T.);
#10655=EDGE_CURVE('',#8510,#8503,#2239,.T.);
#10656=EDGE_CURVE('',#8509,#8511,#2240,.T.);
#10657=EDGE_CURVE('',#8511,#8514,#486,.T.);
#10658=EDGE_CURVE('',#8514,#8510,#2241,.T.);
#10659=EDGE_CURVE('',#8488,#8514,#487,.T.);
#10660=EDGE_CURVE('',#8513,#8514,#2242,.T.);
#10661=EDGE_CURVE('',#8515,#8473,#488,.T.);
#10662=EDGE_CURVE('',#8470,#8515,#2243,.T.);
#10663=EDGE_CURVE('',#8516,#8517,#489,.F.);
#10664=EDGE_CURVE('',#8357,#8516,#490,.F.);
#10665=EDGE_CURVE('',#8517,#8357,#491,.F.);
#10666=EDGE_CURVE('',#8358,#8518,#492,.T.);
#10667=EDGE_CURVE('',#8518,#8398,#493,.T.);
#10668=EDGE_CURVE('',#8516,#8518,#2244,.T.);
#10669=EDGE_CURVE('',#8519,#8517,#2245,.T.);
#10670=EDGE_CURVE('',#8356,#8519,#1819,.T.);
#10671=EDGE_CURVE('',#8520,#8521,#494,.F.);
#10672=EDGE_CURVE('',#8355,#8520,#495,.F.);
#10673=EDGE_CURVE('',#8521,#8355,#496,.F.);
#10674=EDGE_CURVE('',#8520,#8519,#2246,.T.);
#10675=EDGE_CURVE('',#8522,#8521,#2247,.T.);
#10676=EDGE_CURVE('',#8354,#8522,#1820,.T.);
#10677=EDGE_CURVE('',#8353,#8523,#1821,.T.);
#10678=EDGE_CURVE('',#8523,#8522,#2248,.T.);
#10679=EDGE_CURVE('',#8524,#8525,#497,.F.);
#10680=EDGE_CURVE('',#8352,#8524,#498,.F.);
#10681=EDGE_CURVE('',#8525,#8352,#499,.F.);
#10682=EDGE_CURVE('',#8524,#8523,#2249,.T.);
#10683=EDGE_CURVE('',#8526,#8527,#500,.F.);
#10684=EDGE_CURVE('',#8351,#8526,#501,.F.);
#10685=EDGE_CURVE('',#8527,#8351,#502,.F.);
#10686=EDGE_CURVE('',#8526,#8525,#2250,.T.);
#10687=EDGE_CURVE('',#8528,#8529,#503,.F.);
#10688=EDGE_CURVE('',#8350,#8528,#504,.F.);
#10689=EDGE_CURVE('',#8529,#8350,#505,.F.);
#10690=EDGE_CURVE('',#8528,#8527,#2251,.T.);
#10691=EDGE_CURVE('',#8402,#8529,#2252,.T.);
#10692=EDGE_CURVE('',#8530,#8531,#506,.T.);
#10693=EDGE_CURVE('',#8531,#8528,#2253,.T.);
#10694=EDGE_CURVE('',#8529,#8530,#2254,.T.);
#10695=EDGE_CURVE('',#8483,#8530,#507,.T.);
#10696=EDGE_CURVE('',#8530,#8498,#2255,.T.);
#10697=EDGE_CURVE('',#8532,#8533,#508,.T.);
#10698=EDGE_CURVE('',#8533,#8526,#2256,.T.);
#10699=EDGE_CURVE('',#8527,#8532,#2257,.T.);
#10700=EDGE_CURVE('',#8532,#8482,#509,.T.);
#10701=EDGE_CURVE('',#8482,#8533,#510,.T.);
#10702=EDGE_CURVE('',#8534,#8535,#511,.T.);
#10703=EDGE_CURVE('',#8535,#8524,#2258,.T.);
#10704=EDGE_CURVE('',#8525,#8534,#2259,.T.);
#10705=EDGE_CURVE('',#8534,#8481,#512,.T.);
#10706=EDGE_CURVE('',#8481,#8535,#513,.T.);
#10707=EDGE_CURVE('',#8536,#8537,#514,.T.);
#10708=EDGE_CURVE('',#8537,#8520,#2260,.T.);
#10709=EDGE_CURVE('',#8521,#8536,#2261,.T.);
#10710=EDGE_CURVE('',#8536,#8478,#515,.T.);
#10711=EDGE_CURVE('',#8478,#8537,#516,.T.);
#10712=EDGE_CURVE('',#8538,#8539,#517,.T.);
#10713=EDGE_CURVE('',#8539,#8516,#2262,.T.);
#10714=EDGE_CURVE('',#8517,#8538,#2263,.T.);
#10715=EDGE_CURVE('',#8538,#8476,#518,.T.);
#10716=EDGE_CURVE('',#8476,#8539,#519,.T.);
#10717=EDGE_CURVE('',#8397,#8540,#2264,.T.);
#10718=EDGE_CURVE('',#8540,#8515,#520,.T.);
#10719=EDGE_CURVE('',#8515,#8396,#2265,.T.);
#10720=EDGE_CURVE('',#8483,#8531,#521,.T.);
#10721=EDGE_CURVE('',#8540,#8473,#522,.T.);
#10722=EDGE_CURVE('',#8541,#8475,#523,.T.);
#10723=EDGE_CURVE('',#8541,#8539,#2266,.T.);
#10724=EDGE_CURVE('',#8538,#8542,#2267,.T.);
#10725=EDGE_CURVE('',#8477,#8542,#1822,.T.);
#10726=EDGE_CURVE('',#8519,#8542,#2268,.T.);
#10727=EDGE_CURVE('',#8542,#8537,#2269,.T.);
#10728=EDGE_CURVE('',#8536,#8543,#2270,.T.);
#10729=EDGE_CURVE('',#8479,#8543,#1823,.T.);
#10730=EDGE_CURVE('',#8522,#8543,#2271,.T.);
#10731=EDGE_CURVE('',#8523,#8544,#2272,.T.);
#10732=EDGE_CURVE('',#8543,#8544,#2273,.T.);
#10733=EDGE_CURVE('',#8544,#8535,#2274,.T.);
#10734=EDGE_CURVE('',#8480,#8544,#1824,.T.);
#10735=EDGE_CURVE('',#8534,#8533,#2275,.T.);
#10736=EDGE_CURVE('',#8532,#8531,#2276,.T.);
#10737=EDGE_CURVE('',#8540,#8545,#2277,.T.);
#10738=EDGE_CURVE('',#8545,#8474,#524,.T.);
#10739=EDGE_CURVE('',#8545,#8541,#525,.T.);
#10740=EDGE_CURVE('',#8518,#8541,#2278,.T.);
#10741=EDGE_CURVE('',#8398,#8545,#2279,.T.);
#10742=EDGE_CURVE('',#8504,#8512,#526,.T.);
#10743=EDGE_CURVE('',#8507,#8505,#2280,.T.);
#10744=EDGE_CURVE('',#8495,#8378,#527,.T.);
#10745=EDGE_CURVE('',#8490,#8387,#528,.T.);
#10746=EDGE_CURVE('',#8389,#8489,#529,.T.);
#10747=EDGE_CURVE('',#8546,#8491,#530,.T.);
#10748=EDGE_CURVE('',#8389,#8546,#531,.T.);
#10749=EDGE_CURVE('',#8388,#8492,#532,.T.);
#10750=EDGE_CURVE('',#8546,#8388,#2281,.T.);
#10751=EDGE_CURVE('',#8386,#8546,#2282,.T.);
#10752=EDGE_CURVE('',#8286,#8494,#533,.T.);
#10753=EDGE_CURVE('',#8547,#8548,#534,.T.);
#10754=EDGE_CURVE('',#8548,#8493,#535,.T.);
#10755=EDGE_CURVE('',#8548,#8547,#536,.T.);
#10756=EDGE_CURVE('',#8549,#8550,#537,.T.);
#10757=EDGE_CURVE('',#8550,#8549,#538,.T.);
#10758=EDGE_CURVE('',#8550,#8547,#2283,.T.);
#10759=EDGE_CURVE('',#8549,#8382,#539,.T.);
#13539=ORIENTED_EDGE('',*,*,#10244,.T.);
#13540=ORIENTED_EDGE('',*,*,#10245,.T.);
#13541=ORIENTED_EDGE('',*,*,#10246,.T.);
#13542=ORIENTED_EDGE('',*,*,#10247,.T.);
#13543=ORIENTED_EDGE('',*,*,#10245,.F.);
#13544=ORIENTED_EDGE('',*,*,#10248,.T.);
#13545=ORIENTED_EDGE('',*,*,#10249,.F.);
#13546=ORIENTED_EDGE('',*,*,#10250,.F.);
#13547=ORIENTED_EDGE('',*,*,#10251,.T.);
#13548=ORIENTED_EDGE('',*,*,#10246,.F.);
#13549=ORIENTED_EDGE('',*,*,#10247,.F.);
#13550=ORIENTED_EDGE('',*,*,#10251,.F.);
#13551=ORIENTED_EDGE('',*,*,#10244,.F.);
#13552=ORIENTED_EDGE('',*,*,#10252,.T.);
#13553=ORIENTED_EDGE('',*,*,#10253,.F.);
#13554=ORIENTED_EDGE('',*,*,#10254,.F.);
#13555=ORIENTED_EDGE('',*,*,#10252,.F.);
#13556=ORIENTED_EDGE('',*,*,#10248,.F.);
#13557=ORIENTED_EDGE('',*,*,#10255,.T.);
#13558=ORIENTED_EDGE('',*,*,#10256,.T.);
#13559=ORIENTED_EDGE('',*,*,#10257,.T.);
#13560=ORIENTED_EDGE('',*,*,#10258,.T.);
#13561=ORIENTED_EDGE('',*,*,#10257,.F.);
#13562=ORIENTED_EDGE('',*,*,#10259,.T.);
#13563=ORIENTED_EDGE('',*,*,#10260,.T.);
#13564=ORIENTED_EDGE('',*,*,#10255,.F.);
#13565=ORIENTED_EDGE('',*,*,#10261,.T.);
#13566=ORIENTED_EDGE('',*,*,#10262,.T.);
#13567=ORIENTED_EDGE('',*,*,#10260,.F.);
#13568=ORIENTED_EDGE('',*,*,#10263,.T.);
#13569=ORIENTED_EDGE('',*,*,#10264,.F.);
#13570=ORIENTED_EDGE('',*,*,#10265,.T.);
#13571=ORIENTED_EDGE('',*,*,#10259,.F.);
#13572=ORIENTED_EDGE('',*,*,#10266,.T.);
#13573=ORIENTED_EDGE('',*,*,#10267,.T.);
#13574=ORIENTED_EDGE('',*,*,#10268,.T.);
#13575=ORIENTED_EDGE('',*,*,#10256,.F.);
#13576=ORIENTED_EDGE('',*,*,#10269,.F.);
#13577=ORIENTED_EDGE('',*,*,#10270,.F.);
#13578=ORIENTED_EDGE('',*,*,#10266,.F.);
#13579=ORIENTED_EDGE('',*,*,#10271,.T.);
#13580=ORIENTED_EDGE('',*,*,#10272,.T.);
#13581=ORIENTED_EDGE('',*,*,#10273,.T.);
#13582=ORIENTED_EDGE('',*,*,#10274,.T.);
#13583=ORIENTED_EDGE('',*,*,#10273,.F.);
#13584=ORIENTED_EDGE('',*,*,#10275,.T.);
#13585=ORIENTED_EDGE('',*,*,#10276,.T.);
#13586=ORIENTED_EDGE('',*,*,#10271,.F.);
#13587=ORIENTED_EDGE('',*,*,#10264,.T.);
#13588=ORIENTED_EDGE('',*,*,#10277,.T.);
#13589=ORIENTED_EDGE('',*,*,#10277,.F.);
#13590=ORIENTED_EDGE('',*,*,#10278,.T.);
#13591=ORIENTED_EDGE('',*,*,#10279,.F.);
#13592=ORIENTED_EDGE('',*,*,#10280,.T.);
#13593=ORIENTED_EDGE('',*,*,#10258,.F.);
#13594=ORIENTED_EDGE('',*,*,#10265,.F.);
#13595=ORIENTED_EDGE('',*,*,#10274,.F.);
#13596=ORIENTED_EDGE('',*,*,#10281,.F.);
#13597=ORIENTED_EDGE('',*,*,#10282,.T.);
#13598=ORIENTED_EDGE('',*,*,#10283,.T.);
#13599=ORIENTED_EDGE('',*,*,#10284,.T.);
#13600=ORIENTED_EDGE('',*,*,#10285,.T.);
#13601=ORIENTED_EDGE('',*,*,#10284,.F.);
#13602=ORIENTED_EDGE('',*,*,#10279,.T.);
#13603=ORIENTED_EDGE('',*,*,#10286,.T.);
#13604=ORIENTED_EDGE('',*,*,#10282,.F.);
#13605=ORIENTED_EDGE('',*,*,#10287,.T.);
#13606=ORIENTED_EDGE('',*,*,#10288,.T.);
#13607=ORIENTED_EDGE('',*,*,#10286,.F.);
#13608=ORIENTED_EDGE('',*,*,#10289,.T.);
#13609=ORIENTED_EDGE('',*,*,#10290,.F.);
#13610=ORIENTED_EDGE('',*,*,#10291,.T.);
#13611=ORIENTED_EDGE('',*,*,#10272,.F.);
#13612=ORIENTED_EDGE('',*,*,#10280,.F.);
#13613=ORIENTED_EDGE('',*,*,#10283,.F.);
#13614=ORIENTED_EDGE('',*,*,#10292,.F.);
#13615=ORIENTED_EDGE('',*,*,#10293,.T.);
#13616=ORIENTED_EDGE('',*,*,#10294,.T.);
#13617=ORIENTED_EDGE('',*,*,#10295,.T.);
#13618=ORIENTED_EDGE('',*,*,#10296,.T.);
#13619=ORIENTED_EDGE('',*,*,#10295,.F.);
#13620=ORIENTED_EDGE('',*,*,#10297,.T.);
#13621=ORIENTED_EDGE('',*,*,#10298,.T.);
#13622=ORIENTED_EDGE('',*,*,#10293,.F.);
#13623=ORIENTED_EDGE('',*,*,#10290,.T.);
#13624=ORIENTED_EDGE('',*,*,#10299,.T.);
#13625=ORIENTED_EDGE('',*,*,#10299,.F.);
#13626=ORIENTED_EDGE('',*,*,#10300,.T.);
#13627=ORIENTED_EDGE('',*,*,#10301,.T.);
#13628=ORIENTED_EDGE('',*,*,#10302,.T.);
#13629=ORIENTED_EDGE('',*,*,#10285,.F.);
#13630=ORIENTED_EDGE('',*,*,#10291,.F.);
#13631=ORIENTED_EDGE('',*,*,#10296,.F.);
#13632=ORIENTED_EDGE('',*,*,#10303,.F.);
#13633=ORIENTED_EDGE('',*,*,#10304,.T.);
#13634=ORIENTED_EDGE('',*,*,#10305,.T.);
#13635=ORIENTED_EDGE('',*,*,#10306,.T.);
#13636=ORIENTED_EDGE('',*,*,#10307,.T.);
#13637=ORIENTED_EDGE('',*,*,#10306,.F.);
#13638=ORIENTED_EDGE('',*,*,#10308,.T.);
#13639=ORIENTED_EDGE('',*,*,#10309,.T.);
#13640=ORIENTED_EDGE('',*,*,#10304,.F.);
#13641=ORIENTED_EDGE('',*,*,#10310,.T.);
#13642=ORIENTED_EDGE('',*,*,#10311,.T.);
#13643=ORIENTED_EDGE('',*,*,#10311,.F.);
#13644=ORIENTED_EDGE('',*,*,#10312,.T.);
#13645=ORIENTED_EDGE('',*,*,#10313,.F.);
#13646=ORIENTED_EDGE('',*,*,#10314,.T.);
#13647=ORIENTED_EDGE('',*,*,#10310,.F.);
#13648=ORIENTED_EDGE('',*,*,#10315,.T.);
#13649=ORIENTED_EDGE('',*,*,#10316,.F.);
#13650=ORIENTED_EDGE('',*,*,#10317,.T.);
#13651=ORIENTED_EDGE('',*,*,#10307,.F.);
#13652=ORIENTED_EDGE('',*,*,#10318,.F.);
#13653=ORIENTED_EDGE('',*,*,#10319,.F.);
#13654=ORIENTED_EDGE('',*,*,#10315,.F.);
#13655=ORIENTED_EDGE('',*,*,#10320,.T.);
#13656=ORIENTED_EDGE('',*,*,#10321,.T.);
#13657=ORIENTED_EDGE('',*,*,#10322,.T.);
#13658=ORIENTED_EDGE('',*,*,#10323,.T.);
#13659=ORIENTED_EDGE('',*,*,#10322,.F.);
#13660=ORIENTED_EDGE('',*,*,#10313,.T.);
#13661=ORIENTED_EDGE('',*,*,#10324,.T.);
#13662=ORIENTED_EDGE('',*,*,#10320,.F.);
#13663=ORIENTED_EDGE('',*,*,#10325,.T.);
#13664=ORIENTED_EDGE('',*,*,#10326,.T.);
#13665=ORIENTED_EDGE('',*,*,#10324,.F.);
#13666=ORIENTED_EDGE('',*,*,#10327,.T.);
#13667=ORIENTED_EDGE('',*,*,#10328,.F.);
#13668=ORIENTED_EDGE('',*,*,#10329,.T.);
#13669=ORIENTED_EDGE('',*,*,#10305,.F.);
#13670=ORIENTED_EDGE('',*,*,#10314,.F.);
#13671=ORIENTED_EDGE('',*,*,#10321,.F.);
#13672=ORIENTED_EDGE('',*,*,#10330,.F.);
#13673=ORIENTED_EDGE('',*,*,#10331,.T.);
#13674=ORIENTED_EDGE('',*,*,#10332,.T.);
#13675=ORIENTED_EDGE('',*,*,#10333,.T.);
#13676=ORIENTED_EDGE('',*,*,#10334,.T.);
#13677=ORIENTED_EDGE('',*,*,#10332,.F.);
#13678=ORIENTED_EDGE('',*,*,#10335,.F.);
#13679=ORIENTED_EDGE('',*,*,#10336,.F.);
#13680=ORIENTED_EDGE('',*,*,#10337,.F.);
#13681=ORIENTED_EDGE('',*,*,#10338,.F.);
#13682=ORIENTED_EDGE('',*,*,#10339,.F.);
#13683=ORIENTED_EDGE('',*,*,#10340,.F.);
#13684=ORIENTED_EDGE('',*,*,#10341,.F.);
#13685=ORIENTED_EDGE('',*,*,#10342,.F.);
#13686=ORIENTED_EDGE('',*,*,#10343,.F.);
#13687=ORIENTED_EDGE('',*,*,#10344,.F.);
#13688=ORIENTED_EDGE('',*,*,#10345,.F.);
#13689=ORIENTED_EDGE('',*,*,#10346,.F.);
#13690=ORIENTED_EDGE('',*,*,#10347,.F.);
#13691=ORIENTED_EDGE('',*,*,#10348,.F.);
#13692=ORIENTED_EDGE('',*,*,#10349,.F.);
#13693=ORIENTED_EDGE('',*,*,#10350,.F.);
#13694=ORIENTED_EDGE('',*,*,#10351,.F.);
#13695=ORIENTED_EDGE('',*,*,#10352,.F.);
#13696=ORIENTED_EDGE('',*,*,#10353,.F.);
#13697=ORIENTED_EDGE('',*,*,#10354,.F.);
#13698=ORIENTED_EDGE('',*,*,#10355,.F.);
#13699=ORIENTED_EDGE('',*,*,#10356,.F.);
#13700=ORIENTED_EDGE('',*,*,#10357,.F.);
#13701=ORIENTED_EDGE('',*,*,#10358,.F.);
#13702=ORIENTED_EDGE('',*,*,#10359,.F.);
#13703=ORIENTED_EDGE('',*,*,#10360,.F.);
#13704=ORIENTED_EDGE('',*,*,#10361,.F.);
#13705=ORIENTED_EDGE('',*,*,#10362,.F.);
#13706=ORIENTED_EDGE('',*,*,#10363,.F.);
#13707=ORIENTED_EDGE('',*,*,#10364,.F.);
#13708=ORIENTED_EDGE('',*,*,#10365,.F.);
#13709=ORIENTED_EDGE('',*,*,#10366,.F.);
#13710=ORIENTED_EDGE('',*,*,#10367,.F.);
#13711=ORIENTED_EDGE('',*,*,#10368,.F.);
#13712=ORIENTED_EDGE('',*,*,#10369,.F.);
#13713=ORIENTED_EDGE('',*,*,#10370,.F.);
#13714=ORIENTED_EDGE('',*,*,#10371,.F.);
#13715=ORIENTED_EDGE('',*,*,#10372,.F.);
#13716=ORIENTED_EDGE('',*,*,#10373,.F.);
#13717=ORIENTED_EDGE('',*,*,#10374,.F.);
#13718=ORIENTED_EDGE('',*,*,#10375,.F.);
#13719=ORIENTED_EDGE('',*,*,#10376,.F.);
#13720=ORIENTED_EDGE('',*,*,#10377,.F.);
#13721=ORIENTED_EDGE('',*,*,#10378,.F.);
#13722=ORIENTED_EDGE('',*,*,#10379,.F.);
#13723=ORIENTED_EDGE('',*,*,#10380,.F.);
#13724=ORIENTED_EDGE('',*,*,#10381,.F.);
#13725=ORIENTED_EDGE('',*,*,#10331,.F.);
#13726=ORIENTED_EDGE('',*,*,#10334,.F.);
#13727=ORIENTED_EDGE('',*,*,#10382,.T.);
#13728=ORIENTED_EDGE('',*,*,#10383,.F.);
#13729=ORIENTED_EDGE('',*,*,#10384,.F.);
#13730=ORIENTED_EDGE('',*,*,#10382,.F.);
#13731=ORIENTED_EDGE('',*,*,#10333,.F.);
#13732=ORIENTED_EDGE('',*,*,#10359,.T.);
#13733=ORIENTED_EDGE('',*,*,#10385,.T.);
#13734=ORIENTED_EDGE('',*,*,#10386,.T.);
#13735=ORIENTED_EDGE('',*,*,#10387,.T.);
#13736=ORIENTED_EDGE('',*,*,#10385,.F.);
#13737=ORIENTED_EDGE('',*,*,#10387,.F.);
#13738=ORIENTED_EDGE('',*,*,#10388,.T.);
#13739=ORIENTED_EDGE('',*,*,#10389,.F.);
#13740=ORIENTED_EDGE('',*,*,#10390,.F.);
#13741=ORIENTED_EDGE('',*,*,#10388,.F.);
#13742=ORIENTED_EDGE('',*,*,#10386,.F.);
#13743=ORIENTED_EDGE('',*,*,#10381,.T.);
#13744=ORIENTED_EDGE('',*,*,#10391,.T.);
#13745=ORIENTED_EDGE('',*,*,#10249,.T.);
#13746=ORIENTED_EDGE('',*,*,#10250,.T.);
#13747=ORIENTED_EDGE('',*,*,#10391,.F.);
#13748=ORIENTED_EDGE('',*,*,#10392,.T.);
#13749=ORIENTED_EDGE('',*,*,#10393,.T.);
#13750=ORIENTED_EDGE('',*,*,#10394,.T.);
#13751=ORIENTED_EDGE('',*,*,#10360,.T.);
#13752=ORIENTED_EDGE('',*,*,#10395,.T.);
#13753=ORIENTED_EDGE('',*,*,#10361,.T.);
#13754=ORIENTED_EDGE('',*,*,#10394,.F.);
#13755=ORIENTED_EDGE('',*,*,#10396,.T.);
#13756=ORIENTED_EDGE('',*,*,#10397,.T.);
#13757=ORIENTED_EDGE('',*,*,#10362,.T.);
#13758=ORIENTED_EDGE('',*,*,#10395,.F.);
#13759=ORIENTED_EDGE('',*,*,#10398,.T.);
#13760=ORIENTED_EDGE('',*,*,#10392,.F.);
#13761=ORIENTED_EDGE('',*,*,#10363,.T.);
#13762=ORIENTED_EDGE('',*,*,#10397,.F.);
#13763=ORIENTED_EDGE('',*,*,#10399,.T.);
#13764=ORIENTED_EDGE('',*,*,#10396,.F.);
#13765=ORIENTED_EDGE('',*,*,#10400,.T.);
#13766=ORIENTED_EDGE('',*,*,#10401,.F.);
#13767=ORIENTED_EDGE('',*,*,#10402,.F.);
#13768=ORIENTED_EDGE('',*,*,#10393,.F.);
#13769=ORIENTED_EDGE('',*,*,#10403,.T.);
#13770=ORIENTED_EDGE('',*,*,#10404,.F.);
#13771=ORIENTED_EDGE('',*,*,#10400,.F.);
#13772=ORIENTED_EDGE('',*,*,#10325,.F.);
#13773=ORIENTED_EDGE('',*,*,#10405,.T.);
#13774=ORIENTED_EDGE('',*,*,#10406,.T.);
#13775=ORIENTED_EDGE('',*,*,#10364,.T.);
#13776=ORIENTED_EDGE('',*,*,#10308,.F.);
#13777=ORIENTED_EDGE('',*,*,#10330,.T.);
#13778=ORIENTED_EDGE('',*,*,#10326,.F.);
#13779=ORIENTED_EDGE('',*,*,#10371,.T.);
#13780=ORIENTED_EDGE('',*,*,#10407,.T.);
#13781=ORIENTED_EDGE('',*,*,#10408,.T.);
#13782=ORIENTED_EDGE('',*,*,#10409,.T.);
#13783=ORIENTED_EDGE('',*,*,#10309,.F.);
#13784=ORIENTED_EDGE('',*,*,#10370,.T.);
#13785=ORIENTED_EDGE('',*,*,#10407,.F.);
#13786=ORIENTED_EDGE('',*,*,#10318,.T.);
#13787=ORIENTED_EDGE('',*,*,#10406,.F.);
#13788=ORIENTED_EDGE('',*,*,#10410,.T.);
#13789=ORIENTED_EDGE('',*,*,#10411,.T.);
#13790=ORIENTED_EDGE('',*,*,#10323,.F.);
#13791=ORIENTED_EDGE('',*,*,#10329,.F.);
#13792=ORIENTED_EDGE('',*,*,#10412,.F.);
#13793=ORIENTED_EDGE('',*,*,#10405,.F.);
#13794=ORIENTED_EDGE('',*,*,#10409,.F.);
#13795=ORIENTED_EDGE('',*,*,#10413,.T.);
#13796=ORIENTED_EDGE('',*,*,#10414,.T.);
#13797=ORIENTED_EDGE('',*,*,#10319,.T.);
#13798=ORIENTED_EDGE('',*,*,#10408,.F.);
#13799=ORIENTED_EDGE('',*,*,#10369,.T.);
#13800=ORIENTED_EDGE('',*,*,#10415,.T.);
#13801=ORIENTED_EDGE('',*,*,#10416,.T.);
#13802=ORIENTED_EDGE('',*,*,#10417,.T.);
#13803=ORIENTED_EDGE('',*,*,#10335,.T.);
#13804=ORIENTED_EDGE('',*,*,#10418,.T.);
#13805=ORIENTED_EDGE('',*,*,#10419,.T.);
#13806=ORIENTED_EDGE('',*,*,#10418,.F.);
#13807=ORIENTED_EDGE('',*,*,#10420,.T.);
#13808=ORIENTED_EDGE('',*,*,#10421,.T.);
#13809=ORIENTED_EDGE('',*,*,#10420,.F.);
#13810=ORIENTED_EDGE('',*,*,#10358,.T.);
#13811=ORIENTED_EDGE('',*,*,#10422,.T.);
#13812=ORIENTED_EDGE('',*,*,#10423,.T.);
#13813=ORIENTED_EDGE('',*,*,#10424,.F.);
#13814=ORIENTED_EDGE('',*,*,#10425,.F.);
#13815=ORIENTED_EDGE('',*,*,#10426,.F.);
#13816=ORIENTED_EDGE('',*,*,#10427,.T.);
#13817=ORIENTED_EDGE('',*,*,#10428,.T.);
#13818=ORIENTED_EDGE('',*,*,#10429,.T.);
#13819=ORIENTED_EDGE('',*,*,#10427,.F.);
#13820=ORIENTED_EDGE('',*,*,#10347,.T.);
#13821=ORIENTED_EDGE('',*,*,#10425,.T.);
#13822=ORIENTED_EDGE('',*,*,#10430,.T.);
#13823=ORIENTED_EDGE('',*,*,#10431,.F.);
#13824=ORIENTED_EDGE('',*,*,#10432,.F.);
#13825=ORIENTED_EDGE('',*,*,#10433,.F.);
#13826=ORIENTED_EDGE('',*,*,#10432,.T.);
#13827=ORIENTED_EDGE('',*,*,#10434,.T.);
#13828=ORIENTED_EDGE('',*,*,#10426,.T.);
#13829=ORIENTED_EDGE('',*,*,#10346,.T.);
#13830=ORIENTED_EDGE('',*,*,#10435,.F.);
#13831=ORIENTED_EDGE('',*,*,#10436,.F.);
#13832=ORIENTED_EDGE('',*,*,#10437,.F.);
#13833=ORIENTED_EDGE('',*,*,#10436,.T.);
#13834=ORIENTED_EDGE('',*,*,#10438,.T.);
#13835=ORIENTED_EDGE('',*,*,#10433,.T.);
#13836=ORIENTED_EDGE('',*,*,#10345,.T.);
#13837=ORIENTED_EDGE('',*,*,#10439,.T.);
#13838=ORIENTED_EDGE('',*,*,#10440,.T.);
#13839=ORIENTED_EDGE('',*,*,#10437,.T.);
#13840=ORIENTED_EDGE('',*,*,#10344,.T.);
#13841=ORIENTED_EDGE('',*,*,#10439,.F.);
#13842=ORIENTED_EDGE('',*,*,#10441,.T.);
#13843=ORIENTED_EDGE('',*,*,#10442,.T.);
#13844=ORIENTED_EDGE('',*,*,#10443,.T.);
#13845=ORIENTED_EDGE('',*,*,#10444,.T.);
#13846=ORIENTED_EDGE('',*,*,#10435,.T.);
#13847=ORIENTED_EDGE('',*,*,#10445,.T.);
#13848=ORIENTED_EDGE('',*,*,#10443,.F.);
#13849=ORIENTED_EDGE('',*,*,#10446,.T.);
#13850=ORIENTED_EDGE('',*,*,#10447,.T.);
#13851=ORIENTED_EDGE('',*,*,#10448,.T.);
#13852=ORIENTED_EDGE('',*,*,#10449,.T.);
#13853=ORIENTED_EDGE('',*,*,#10431,.T.);
#13854=ORIENTED_EDGE('',*,*,#10450,.T.);
#13855=ORIENTED_EDGE('',*,*,#10448,.F.);
#13856=ORIENTED_EDGE('',*,*,#10451,.T.);
#13857=ORIENTED_EDGE('',*,*,#10452,.T.);
#13858=ORIENTED_EDGE('',*,*,#10453,.T.);
#13859=ORIENTED_EDGE('',*,*,#10454,.T.);
#13860=ORIENTED_EDGE('',*,*,#10424,.T.);
#13861=ORIENTED_EDGE('',*,*,#10455,.T.);
#13862=ORIENTED_EDGE('',*,*,#10453,.F.);
#13863=ORIENTED_EDGE('',*,*,#10456,.T.);
#13864=ORIENTED_EDGE('',*,*,#10457,.T.);
#13865=ORIENTED_EDGE('',*,*,#10455,.F.);
#13866=ORIENTED_EDGE('',*,*,#10434,.F.);
#13867=ORIENTED_EDGE('',*,*,#10449,.F.);
#13868=ORIENTED_EDGE('',*,*,#10458,.F.);
#13869=ORIENTED_EDGE('',*,*,#10450,.F.);
#13870=ORIENTED_EDGE('',*,*,#10438,.F.);
#13871=ORIENTED_EDGE('',*,*,#10444,.F.);
#13872=ORIENTED_EDGE('',*,*,#10459,.F.);
#13873=ORIENTED_EDGE('',*,*,#10451,.F.);
#13874=ORIENTED_EDGE('',*,*,#10459,.T.);
#13875=ORIENTED_EDGE('',*,*,#10447,.F.);
#13876=ORIENTED_EDGE('',*,*,#10460,.T.);
#13877=ORIENTED_EDGE('',*,*,#10446,.F.);
#13878=ORIENTED_EDGE('',*,*,#10461,.T.);
#13879=ORIENTED_EDGE('',*,*,#10462,.F.);
#13880=ORIENTED_EDGE('',*,*,#10463,.T.);
#13881=ORIENTED_EDGE('',*,*,#10445,.F.);
#13882=ORIENTED_EDGE('',*,*,#10440,.F.);
#13883=ORIENTED_EDGE('',*,*,#10464,.F.);
#13884=ORIENTED_EDGE('',*,*,#10461,.F.);
#13885=ORIENTED_EDGE('',*,*,#10465,.F.);
#13886=ORIENTED_EDGE('',*,*,#10466,.F.);
#13887=ORIENTED_EDGE('',*,*,#10467,.F.);
#13888=ORIENTED_EDGE('',*,*,#10468,.T.);
#13889=ORIENTED_EDGE('',*,*,#10469,.T.);
#13890=ORIENTED_EDGE('',*,*,#10470,.T.);
#13891=ORIENTED_EDGE('',*,*,#10468,.F.);
#13892=ORIENTED_EDGE('',*,*,#10471,.T.);
#13893=ORIENTED_EDGE('',*,*,#10466,.T.);
#13894=ORIENTED_EDGE('',*,*,#10472,.T.);
#13895=ORIENTED_EDGE('',*,*,#10473,.T.);
#13896=ORIENTED_EDGE('',*,*,#10373,.T.);
#13897=ORIENTED_EDGE('',*,*,#10467,.T.);
#13898=ORIENTED_EDGE('',*,*,#10474,.T.);
#13899=ORIENTED_EDGE('',*,*,#10473,.F.);
#13900=ORIENTED_EDGE('',*,*,#10475,.T.);
#13901=ORIENTED_EDGE('',*,*,#10476,.T.);
#13902=ORIENTED_EDGE('',*,*,#10477,.T.);
#13903=ORIENTED_EDGE('',*,*,#10478,.T.);
#13904=ORIENTED_EDGE('',*,*,#10465,.T.);
#13905=ORIENTED_EDGE('',*,*,#10380,.T.);
#13906=ORIENTED_EDGE('',*,*,#10297,.F.);
#13907=ORIENTED_EDGE('',*,*,#10479,.T.);
#13908=ORIENTED_EDGE('',*,*,#10480,.T.);
#13909=ORIENTED_EDGE('',*,*,#10379,.T.);
#13910=ORIENTED_EDGE('',*,*,#10287,.F.);
#13911=ORIENTED_EDGE('',*,*,#10303,.T.);
#13912=ORIENTED_EDGE('',*,*,#10298,.F.);
#13913=ORIENTED_EDGE('',*,*,#10378,.T.);
#13914=ORIENTED_EDGE('',*,*,#10275,.F.);
#13915=ORIENTED_EDGE('',*,*,#10292,.T.);
#13916=ORIENTED_EDGE('',*,*,#10288,.F.);
#13917=ORIENTED_EDGE('',*,*,#10377,.T.);
#13918=ORIENTED_EDGE('',*,*,#10261,.F.);
#13919=ORIENTED_EDGE('',*,*,#10281,.T.);
#13920=ORIENTED_EDGE('',*,*,#10276,.F.);
#13921=ORIENTED_EDGE('',*,*,#10376,.T.);
#13922=ORIENTED_EDGE('',*,*,#10481,.T.);
#13923=ORIENTED_EDGE('',*,*,#10482,.T.);
#13924=ORIENTED_EDGE('',*,*,#10483,.T.);
#13925=ORIENTED_EDGE('',*,*,#10262,.F.);
#13926=ORIENTED_EDGE('',*,*,#10375,.T.);
#13927=ORIENTED_EDGE('',*,*,#10481,.F.);
#13928=ORIENTED_EDGE('',*,*,#10269,.T.);
#13929=ORIENTED_EDGE('',*,*,#10480,.F.);
#13930=ORIENTED_EDGE('',*,*,#10484,.T.);
#13931=ORIENTED_EDGE('',*,*,#10477,.F.);
#13932=ORIENTED_EDGE('',*,*,#10470,.F.);
#13933=ORIENTED_EDGE('',*,*,#10485,.T.);
#13934=ORIENTED_EDGE('',*,*,#10486,.F.);
#13935=ORIENTED_EDGE('',*,*,#10487,.T.);
#13936=ORIENTED_EDGE('',*,*,#10469,.F.);
#13937=ORIENTED_EDGE('',*,*,#10488,.T.);
#13938=ORIENTED_EDGE('',*,*,#10489,.F.);
#13939=ORIENTED_EDGE('',*,*,#10490,.T.);
#13940=ORIENTED_EDGE('',*,*,#10472,.F.);
#13941=ORIENTED_EDGE('',*,*,#10478,.F.);
#13942=ORIENTED_EDGE('',*,*,#10491,.F.);
#13943=ORIENTED_EDGE('',*,*,#10488,.F.);
#13944=ORIENTED_EDGE('',*,*,#10484,.F.);
#13945=ORIENTED_EDGE('',*,*,#10492,.T.);
#13946=ORIENTED_EDGE('',*,*,#10493,.T.);
#13947=ORIENTED_EDGE('',*,*,#10491,.T.);
#13948=ORIENTED_EDGE('',*,*,#10294,.F.);
#13949=ORIENTED_EDGE('',*,*,#10302,.F.);
#13950=ORIENTED_EDGE('',*,*,#10492,.F.);
#13951=ORIENTED_EDGE('',*,*,#10479,.F.);
#13952=ORIENTED_EDGE('',*,*,#10483,.F.);
#13953=ORIENTED_EDGE('',*,*,#10494,.T.);
#13954=ORIENTED_EDGE('',*,*,#10495,.T.);
#13955=ORIENTED_EDGE('',*,*,#10270,.T.);
#13956=ORIENTED_EDGE('',*,*,#10372,.T.);
#13957=ORIENTED_EDGE('',*,*,#10496,.T.);
#13958=ORIENTED_EDGE('',*,*,#10497,.T.);
#13959=ORIENTED_EDGE('',*,*,#10498,.T.);
#13960=ORIENTED_EDGE('',*,*,#10496,.F.);
#13961=ORIENTED_EDGE('',*,*,#10498,.F.);
#13962=ORIENTED_EDGE('',*,*,#10499,.T.);
#13963=ORIENTED_EDGE('',*,*,#10500,.F.);
#13964=ORIENTED_EDGE('',*,*,#10501,.F.);
#13965=ORIENTED_EDGE('',*,*,#10499,.F.);
#13966=ORIENTED_EDGE('',*,*,#10497,.F.);
#13967=ORIENTED_EDGE('',*,*,#10502,.F.);
#13968=ORIENTED_EDGE('',*,*,#10503,.F.);
#13969=ORIENTED_EDGE('',*,*,#10504,.F.);
#13970=ORIENTED_EDGE('',*,*,#10441,.F.);
#13971=ORIENTED_EDGE('',*,*,#10343,.T.);
#13972=ORIENTED_EDGE('',*,*,#10503,.T.);
#13973=ORIENTED_EDGE('',*,*,#10505,.T.);
#13974=ORIENTED_EDGE('',*,*,#10506,.F.);
#13975=ORIENTED_EDGE('',*,*,#10507,.F.);
#13976=ORIENTED_EDGE('',*,*,#10508,.F.);
#13977=ORIENTED_EDGE('',*,*,#10507,.T.);
#13978=ORIENTED_EDGE('',*,*,#10509,.T.);
#13979=ORIENTED_EDGE('',*,*,#10504,.T.);
#13980=ORIENTED_EDGE('',*,*,#10342,.T.);
#13981=ORIENTED_EDGE('',*,*,#10510,.F.);
#13982=ORIENTED_EDGE('',*,*,#10511,.F.);
#13983=ORIENTED_EDGE('',*,*,#10512,.F.);
#13984=ORIENTED_EDGE('',*,*,#10511,.T.);
#13985=ORIENTED_EDGE('',*,*,#10513,.T.);
#13986=ORIENTED_EDGE('',*,*,#10508,.T.);
#13987=ORIENTED_EDGE('',*,*,#10341,.T.);
#13988=ORIENTED_EDGE('',*,*,#10514,.F.);
#13989=ORIENTED_EDGE('',*,*,#10515,.F.);
#13990=ORIENTED_EDGE('',*,*,#10516,.F.);
#13991=ORIENTED_EDGE('',*,*,#10515,.T.);
#13992=ORIENTED_EDGE('',*,*,#10517,.T.);
#13993=ORIENTED_EDGE('',*,*,#10512,.T.);
#13994=ORIENTED_EDGE('',*,*,#10340,.T.);
#13995=ORIENTED_EDGE('',*,*,#10518,.T.);
#13996=ORIENTED_EDGE('',*,*,#10516,.T.);
#13997=ORIENTED_EDGE('',*,*,#10339,.T.);
#13998=ORIENTED_EDGE('',*,*,#10519,.T.);
#13999=ORIENTED_EDGE('',*,*,#10338,.T.);
#14000=ORIENTED_EDGE('',*,*,#10520,.T.);
#14001=ORIENTED_EDGE('',*,*,#10521,.T.);
#14002=ORIENTED_EDGE('',*,*,#10519,.F.);
#14003=ORIENTED_EDGE('',*,*,#10522,.F.);
#14004=ORIENTED_EDGE('',*,*,#10523,.F.);
#14005=ORIENTED_EDGE('',*,*,#10524,.F.);
#14006=ORIENTED_EDGE('',*,*,#10337,.T.);
#14007=ORIENTED_EDGE('',*,*,#10523,.T.);
#14008=ORIENTED_EDGE('',*,*,#10525,.T.);
#14009=ORIENTED_EDGE('',*,*,#10520,.F.);
#14010=ORIENTED_EDGE('',*,*,#10526,.T.);
#14011=ORIENTED_EDGE('',*,*,#10524,.T.);
#14012=ORIENTED_EDGE('',*,*,#10336,.T.);
#14013=ORIENTED_EDGE('',*,*,#10417,.F.);
#14014=ORIENTED_EDGE('',*,*,#10527,.T.);
#14015=ORIENTED_EDGE('',*,*,#10528,.T.);
#14016=ORIENTED_EDGE('',*,*,#10522,.T.);
#14017=ORIENTED_EDGE('',*,*,#10529,.T.);
#14018=ORIENTED_EDGE('',*,*,#10527,.F.);
#14019=ORIENTED_EDGE('',*,*,#10530,.T.);
#14020=ORIENTED_EDGE('',*,*,#10531,.T.);
#14021=ORIENTED_EDGE('',*,*,#10532,.T.);
#14022=ORIENTED_EDGE('',*,*,#10533,.T.);
#14023=ORIENTED_EDGE('',*,*,#10514,.T.);
#14024=ORIENTED_EDGE('',*,*,#10534,.T.);
#14025=ORIENTED_EDGE('',*,*,#10532,.F.);
#14026=ORIENTED_EDGE('',*,*,#10535,.T.);
#14027=ORIENTED_EDGE('',*,*,#10536,.T.);
#14028=ORIENTED_EDGE('',*,*,#10537,.T.);
#14029=ORIENTED_EDGE('',*,*,#10538,.T.);
#14030=ORIENTED_EDGE('',*,*,#10510,.T.);
#14031=ORIENTED_EDGE('',*,*,#10539,.T.);
#14032=ORIENTED_EDGE('',*,*,#10537,.F.);
#14033=ORIENTED_EDGE('',*,*,#10540,.T.);
#14034=ORIENTED_EDGE('',*,*,#10541,.T.);
#14035=ORIENTED_EDGE('',*,*,#10542,.T.);
#14036=ORIENTED_EDGE('',*,*,#10543,.T.);
#14037=ORIENTED_EDGE('',*,*,#10506,.T.);
#14038=ORIENTED_EDGE('',*,*,#10544,.T.);
#14039=ORIENTED_EDGE('',*,*,#10542,.F.);
#14040=ORIENTED_EDGE('',*,*,#10545,.T.);
#14041=ORIENTED_EDGE('',*,*,#10546,.T.);
#14042=ORIENTED_EDGE('',*,*,#10547,.T.);
#14043=ORIENTED_EDGE('',*,*,#10548,.T.);
#14044=ORIENTED_EDGE('',*,*,#10502,.T.);
#14045=ORIENTED_EDGE('',*,*,#10549,.T.);
#14046=ORIENTED_EDGE('',*,*,#10547,.F.);
#14047=ORIENTED_EDGE('',*,*,#10550,.T.);
#14048=ORIENTED_EDGE('',*,*,#10551,.T.);
#14049=ORIENTED_EDGE('',*,*,#10442,.F.);
#14050=ORIENTED_EDGE('',*,*,#10552,.T.);
#14051=ORIENTED_EDGE('',*,*,#10553,.T.);
#14052=ORIENTED_EDGE('',*,*,#10464,.T.);
#14053=ORIENTED_EDGE('',*,*,#10553,.F.);
#14054=ORIENTED_EDGE('',*,*,#10554,.T.);
#14055=ORIENTED_EDGE('',*,*,#10462,.T.);
#14056=ORIENTED_EDGE('',*,*,#10544,.F.);
#14057=ORIENTED_EDGE('',*,*,#10513,.F.);
#14058=ORIENTED_EDGE('',*,*,#10538,.F.);
#14059=ORIENTED_EDGE('',*,*,#10555,.F.);
#14060=ORIENTED_EDGE('',*,*,#10546,.F.);
#14061=ORIENTED_EDGE('',*,*,#10556,.T.);
#14062=ORIENTED_EDGE('',*,*,#10550,.F.);
#14063=ORIENTED_EDGE('',*,*,#10557,.T.);
#14064=ORIENTED_EDGE('',*,*,#10545,.F.);
#14065=ORIENTED_EDGE('',*,*,#10555,.T.);
#14066=ORIENTED_EDGE('',*,*,#10541,.F.);
#14067=ORIENTED_EDGE('',*,*,#10558,.T.);
#14068=ORIENTED_EDGE('',*,*,#10539,.F.);
#14069=ORIENTED_EDGE('',*,*,#10517,.F.);
#14070=ORIENTED_EDGE('',*,*,#10533,.F.);
#14071=ORIENTED_EDGE('',*,*,#10559,.F.);
#14072=ORIENTED_EDGE('',*,*,#10540,.F.);
#14073=ORIENTED_EDGE('',*,*,#10559,.T.);
#14074=ORIENTED_EDGE('',*,*,#10536,.F.);
#14075=ORIENTED_EDGE('',*,*,#10560,.T.);
#14076=ORIENTED_EDGE('',*,*,#10535,.F.);
#14077=ORIENTED_EDGE('',*,*,#10561,.T.);
#14078=ORIENTED_EDGE('',*,*,#10562,.F.);
#14079=ORIENTED_EDGE('',*,*,#10563,.T.);
#14080=ORIENTED_EDGE('',*,*,#10534,.F.);
#14081=ORIENTED_EDGE('',*,*,#10518,.F.);
#14082=ORIENTED_EDGE('',*,*,#10564,.T.);
#14083=ORIENTED_EDGE('',*,*,#10561,.F.);
#14084=ORIENTED_EDGE('',*,*,#10521,.F.);
#14085=ORIENTED_EDGE('',*,*,#10565,.T.);
#14086=ORIENTED_EDGE('',*,*,#10566,.F.);
#14087=ORIENTED_EDGE('',*,*,#10564,.F.);
#14088=ORIENTED_EDGE('',*,*,#10525,.F.);
#14089=ORIENTED_EDGE('',*,*,#10528,.F.);
#14090=ORIENTED_EDGE('',*,*,#10567,.F.);
#14091=ORIENTED_EDGE('',*,*,#10565,.F.);
#14092=ORIENTED_EDGE('',*,*,#10531,.F.);
#14093=ORIENTED_EDGE('',*,*,#10568,.T.);
#14094=ORIENTED_EDGE('',*,*,#10569,.T.);
#14095=ORIENTED_EDGE('',*,*,#10567,.T.);
#14096=ORIENTED_EDGE('',*,*,#10530,.F.);
#14097=ORIENTED_EDGE('',*,*,#10570,.T.);
#14098=ORIENTED_EDGE('',*,*,#10571,.T.);
#14099=ORIENTED_EDGE('',*,*,#10572,.T.);
#14100=ORIENTED_EDGE('',*,*,#10529,.F.);
#14101=ORIENTED_EDGE('',*,*,#10526,.F.);
#14102=ORIENTED_EDGE('',*,*,#10573,.T.);
#14103=ORIENTED_EDGE('',*,*,#10570,.F.);
#14104=ORIENTED_EDGE('',*,*,#10574,.T.);
#14105=ORIENTED_EDGE('',*,*,#10575,.T.);
#14106=ORIENTED_EDGE('',*,*,#10500,.T.);
#14107=ORIENTED_EDGE('',*,*,#10501,.T.);
#14108=ORIENTED_EDGE('',*,*,#10575,.F.);
#14109=ORIENTED_EDGE('',*,*,#10576,.F.);
#14110=ORIENTED_EDGE('',*,*,#10577,.F.);
#14111=ORIENTED_EDGE('',*,*,#10578,.F.);
#14112=ORIENTED_EDGE('',*,*,#10579,.F.);
#14113=ORIENTED_EDGE('',*,*,#10580,.F.);
#14114=ORIENTED_EDGE('',*,*,#10581,.F.);
#14115=ORIENTED_EDGE('',*,*,#10582,.F.);
#14116=ORIENTED_EDGE('',*,*,#10583,.F.);
#14117=ORIENTED_EDGE('',*,*,#10584,.F.);
#14118=ORIENTED_EDGE('',*,*,#10585,.F.);
#14119=ORIENTED_EDGE('',*,*,#10586,.F.);
#14120=ORIENTED_EDGE('',*,*,#10587,.F.);
#14121=ORIENTED_EDGE('',*,*,#10588,.F.);
#14122=ORIENTED_EDGE('',*,*,#10589,.F.);
#14123=ORIENTED_EDGE('',*,*,#10460,.F.);
#14124=ORIENTED_EDGE('',*,*,#10463,.F.);
#14125=ORIENTED_EDGE('',*,*,#10590,.F.);
#14126=ORIENTED_EDGE('',*,*,#10556,.F.);
#14127=ORIENTED_EDGE('',*,*,#10558,.F.);
#14128=ORIENTED_EDGE('',*,*,#10560,.F.);
#14129=ORIENTED_EDGE('',*,*,#10563,.F.);
#14130=ORIENTED_EDGE('',*,*,#10591,.F.);
#14131=ORIENTED_EDGE('',*,*,#10568,.F.);
#14132=ORIENTED_EDGE('',*,*,#10572,.F.);
#14133=ORIENTED_EDGE('',*,*,#10592,.F.);
#14134=ORIENTED_EDGE('',*,*,#10593,.F.);
#14135=ORIENTED_EDGE('',*,*,#10594,.F.);
#14136=ORIENTED_EDGE('',*,*,#10595,.F.);
#14137=ORIENTED_EDGE('',*,*,#10596,.F.);
#14138=ORIENTED_EDGE('',*,*,#10327,.F.);
#14139=ORIENTED_EDGE('',*,*,#10312,.F.);
#14140=ORIENTED_EDGE('',*,*,#10317,.F.);
#14141=ORIENTED_EDGE('',*,*,#10597,.F.);
#14142=ORIENTED_EDGE('',*,*,#10598,.F.);
#14143=ORIENTED_EDGE('',*,*,#10599,.F.);
#14144=ORIENTED_EDGE('',*,*,#10600,.F.);
#14145=ORIENTED_EDGE('',*,*,#10601,.F.);
#14146=ORIENTED_EDGE('',*,*,#10300,.F.);
#14147=ORIENTED_EDGE('',*,*,#10289,.F.);
#14148=ORIENTED_EDGE('',*,*,#10278,.F.);
#14149=ORIENTED_EDGE('',*,*,#10263,.F.);
#14150=ORIENTED_EDGE('',*,*,#10268,.F.);
#14151=ORIENTED_EDGE('',*,*,#10602,.F.);
#14152=ORIENTED_EDGE('',*,*,#10485,.F.);
#14153=ORIENTED_EDGE('',*,*,#10490,.F.);
#14154=ORIENTED_EDGE('',*,*,#10603,.F.);
#14155=ORIENTED_EDGE('',*,*,#10604,.F.);
#14156=ORIENTED_EDGE('',*,*,#10574,.F.);
#14157=ORIENTED_EDGE('',*,*,#10495,.F.);
#14158=ORIENTED_EDGE('',*,*,#10605,.F.);
#14159=ORIENTED_EDGE('',*,*,#10267,.F.);
#14160=ORIENTED_EDGE('',*,*,#10606,.T.);
#14161=ORIENTED_EDGE('',*,*,#10602,.T.);
#14162=ORIENTED_EDGE('',*,*,#10605,.T.);
#14163=ORIENTED_EDGE('',*,*,#10607,.T.);
#14164=ORIENTED_EDGE('',*,*,#10476,.F.);
#14165=ORIENTED_EDGE('',*,*,#10608,.T.);
#14166=ORIENTED_EDGE('',*,*,#10482,.F.);
#14167=ORIENTED_EDGE('',*,*,#10374,.T.);
#14168=ORIENTED_EDGE('',*,*,#10475,.F.);
#14169=ORIENTED_EDGE('',*,*,#10609,.T.);
#14170=ORIENTED_EDGE('',*,*,#10610,.T.);
#14171=ORIENTED_EDGE('',*,*,#10611,.T.);
#14172=ORIENTED_EDGE('',*,*,#10610,.F.);
#14173=ORIENTED_EDGE('',*,*,#10486,.T.);
#14174=ORIENTED_EDGE('',*,*,#10606,.F.);
#14175=ORIENTED_EDGE('',*,*,#10301,.F.);
#14176=ORIENTED_EDGE('',*,*,#10489,.T.);
#14177=ORIENTED_EDGE('',*,*,#10493,.F.);
#14178=ORIENTED_EDGE('',*,*,#10471,.F.);
#14179=ORIENTED_EDGE('',*,*,#10487,.F.);
#14180=ORIENTED_EDGE('',*,*,#10609,.F.);
#14181=ORIENTED_EDGE('',*,*,#10474,.F.);
#14182=ORIENTED_EDGE('',*,*,#10607,.F.);
#14183=ORIENTED_EDGE('',*,*,#10494,.F.);
#14184=ORIENTED_EDGE('',*,*,#10608,.F.);
#14185=ORIENTED_EDGE('',*,*,#10611,.F.);
#14186=ORIENTED_EDGE('',*,*,#10591,.T.);
#14187=ORIENTED_EDGE('',*,*,#10562,.T.);
#14188=ORIENTED_EDGE('',*,*,#10566,.T.);
#14189=ORIENTED_EDGE('',*,*,#10569,.F.);
#14190=ORIENTED_EDGE('',*,*,#10551,.F.);
#14191=ORIENTED_EDGE('',*,*,#10590,.T.);
#14192=ORIENTED_EDGE('',*,*,#10554,.F.);
#14193=ORIENTED_EDGE('',*,*,#10612,.T.);
#14194=ORIENTED_EDGE('',*,*,#10456,.F.);
#14195=ORIENTED_EDGE('',*,*,#10458,.T.);
#14196=ORIENTED_EDGE('',*,*,#10452,.F.);
#14197=ORIENTED_EDGE('',*,*,#10589,.T.);
#14198=ORIENTED_EDGE('',*,*,#10613,.T.);
#14199=ORIENTED_EDGE('',*,*,#10614,.T.);
#14200=ORIENTED_EDGE('',*,*,#10615,.T.);
#14201=ORIENTED_EDGE('',*,*,#10457,.F.);
#14202=ORIENTED_EDGE('',*,*,#10588,.T.);
#14203=ORIENTED_EDGE('',*,*,#10613,.F.);
#14204=ORIENTED_EDGE('',*,*,#10616,.T.);
#14205=ORIENTED_EDGE('',*,*,#10543,.F.);
#14206=ORIENTED_EDGE('',*,*,#10557,.F.);
#14207=ORIENTED_EDGE('',*,*,#10549,.F.);
#14208=ORIENTED_EDGE('',*,*,#10509,.F.);
#14209=ORIENTED_EDGE('',*,*,#10548,.F.);
#14210=ORIENTED_EDGE('',*,*,#10612,.F.);
#14211=ORIENTED_EDGE('',*,*,#10552,.F.);
#14212=ORIENTED_EDGE('',*,*,#10505,.F.);
#14213=ORIENTED_EDGE('',*,*,#10454,.F.);
#14214=ORIENTED_EDGE('',*,*,#10616,.F.);
#14215=ORIENTED_EDGE('',*,*,#10617,.F.);
#14216=ORIENTED_EDGE('',*,*,#10430,.F.);
#14217=ORIENTED_EDGE('',*,*,#10428,.F.);
#14218=ORIENTED_EDGE('',*,*,#10617,.T.);
#14219=ORIENTED_EDGE('',*,*,#10615,.F.);
#14220=ORIENTED_EDGE('',*,*,#10618,.T.);
#14221=ORIENTED_EDGE('',*,*,#10619,.F.);
#14222=ORIENTED_EDGE('',*,*,#10415,.F.);
#14223=ORIENTED_EDGE('',*,*,#10620,.F.);
#14224=ORIENTED_EDGE('',*,*,#10621,.F.);
#14225=ORIENTED_EDGE('',*,*,#10622,.F.);
#14226=ORIENTED_EDGE('',*,*,#10623,.F.);
#14227=ORIENTED_EDGE('',*,*,#10620,.T.);
#14228=ORIENTED_EDGE('',*,*,#10368,.T.);
#14229=ORIENTED_EDGE('',*,*,#10622,.T.);
#14230=ORIENTED_EDGE('',*,*,#10624,.T.);
#14231=ORIENTED_EDGE('',*,*,#10625,.T.);
#14232=ORIENTED_EDGE('',*,*,#10626,.T.);
#14233=ORIENTED_EDGE('',*,*,#10627,.T.);
#14234=ORIENTED_EDGE('',*,*,#10625,.F.);
#14235=ORIENTED_EDGE('',*,*,#10628,.T.);
#14236=ORIENTED_EDGE('',*,*,#10623,.T.);
#14237=ORIENTED_EDGE('',*,*,#10367,.T.);
#14238=ORIENTED_EDGE('',*,*,#10629,.T.);
#14239=ORIENTED_EDGE('',*,*,#10630,.T.);
#14240=ORIENTED_EDGE('',*,*,#10621,.T.);
#14241=ORIENTED_EDGE('',*,*,#10631,.T.);
#14242=ORIENTED_EDGE('',*,*,#10629,.F.);
#14243=ORIENTED_EDGE('',*,*,#10632,.T.);
#14244=ORIENTED_EDGE('',*,*,#10633,.T.);
#14245=ORIENTED_EDGE('',*,*,#10634,.T.);
#14246=ORIENTED_EDGE('',*,*,#10635,.T.);
#14247=ORIENTED_EDGE('',*,*,#10636,.T.);
#14248=ORIENTED_EDGE('',*,*,#10634,.F.);
#14249=ORIENTED_EDGE('',*,*,#10637,.T.);
#14250=ORIENTED_EDGE('',*,*,#10619,.T.);
#14251=ORIENTED_EDGE('',*,*,#10638,.T.);
#14252=ORIENTED_EDGE('',*,*,#10414,.F.);
#14253=ORIENTED_EDGE('',*,*,#10639,.T.);
#14254=ORIENTED_EDGE('',*,*,#10316,.T.);
#14255=ORIENTED_EDGE('',*,*,#10413,.F.);
#14256=ORIENTED_EDGE('',*,*,#10416,.F.);
#14257=ORIENTED_EDGE('',*,*,#10637,.F.);
#14258=ORIENTED_EDGE('',*,*,#10640,.F.);
#14259=ORIENTED_EDGE('',*,*,#10639,.F.);
#14260=ORIENTED_EDGE('',*,*,#10640,.T.);
#14261=ORIENTED_EDGE('',*,*,#10636,.F.);
#14262=ORIENTED_EDGE('',*,*,#10592,.T.);
#14263=ORIENTED_EDGE('',*,*,#10641,.T.);
#14264=ORIENTED_EDGE('',*,*,#10328,.T.);
#14265=ORIENTED_EDGE('',*,*,#10642,.T.);
#14266=ORIENTED_EDGE('',*,*,#10410,.F.);
#14267=ORIENTED_EDGE('',*,*,#10412,.T.);
#14268=ORIENTED_EDGE('',*,*,#10641,.F.);
#14269=ORIENTED_EDGE('',*,*,#10643,.T.);
#14270=ORIENTED_EDGE('',*,*,#10411,.F.);
#14271=ORIENTED_EDGE('',*,*,#10644,.T.);
#14272=ORIENTED_EDGE('',*,*,#10645,.T.);
#14273=ORIENTED_EDGE('',*,*,#10365,.T.);
#14274=ORIENTED_EDGE('',*,*,#10645,.F.);
#14275=ORIENTED_EDGE('',*,*,#10646,.T.);
#14276=ORIENTED_EDGE('',*,*,#10647,.T.);
#14277=ORIENTED_EDGE('',*,*,#10642,.F.);
#14278=ORIENTED_EDGE('',*,*,#10596,.T.);
#14279=ORIENTED_EDGE('',*,*,#10648,.F.);
#14280=ORIENTED_EDGE('',*,*,#10649,.T.);
#14281=ORIENTED_EDGE('',*,*,#10650,.T.);
#14282=ORIENTED_EDGE('',*,*,#10651,.T.);
#14283=ORIENTED_EDGE('',*,*,#10652,.T.);
#14284=ORIENTED_EDGE('',*,*,#10627,.F.);
#14285=ORIENTED_EDGE('',*,*,#10653,.T.);
#14286=ORIENTED_EDGE('',*,*,#10650,.F.);
#14287=ORIENTED_EDGE('',*,*,#10654,.T.);
#14288=ORIENTED_EDGE('',*,*,#10626,.F.);
#14289=ORIENTED_EDGE('',*,*,#10366,.T.);
#14290=ORIENTED_EDGE('',*,*,#10647,.F.);
#14291=ORIENTED_EDGE('',*,*,#10655,.T.);
#14292=ORIENTED_EDGE('',*,*,#10646,.F.);
#14293=ORIENTED_EDGE('',*,*,#10656,.T.);
#14294=ORIENTED_EDGE('',*,*,#10657,.T.);
#14295=ORIENTED_EDGE('',*,*,#10658,.T.);
#14296=ORIENTED_EDGE('',*,*,#10657,.F.);
#14297=ORIENTED_EDGE('',*,*,#10648,.T.);
#14298=ORIENTED_EDGE('',*,*,#10659,.T.);
#14299=ORIENTED_EDGE('',*,*,#10653,.F.);
#14300=ORIENTED_EDGE('',*,*,#10655,.F.);
#14301=ORIENTED_EDGE('',*,*,#10658,.F.);
#14302=ORIENTED_EDGE('',*,*,#10660,.F.);
#14303=ORIENTED_EDGE('',*,*,#10643,.F.);
#14304=ORIENTED_EDGE('',*,*,#10649,.F.);
#14305=ORIENTED_EDGE('',*,*,#10656,.F.);
#14306=ORIENTED_EDGE('',*,*,#10644,.F.);
#14307=ORIENTED_EDGE('',*,*,#10661,.T.);
#14308=ORIENTED_EDGE('',*,*,#10576,.T.);
#14309=ORIENTED_EDGE('',*,*,#10571,.F.);
#14310=ORIENTED_EDGE('',*,*,#10662,.T.);
#14311=ORIENTED_EDGE('',*,*,#10663,.F.);
#14312=ORIENTED_EDGE('',*,*,#10664,.F.);
#14313=ORIENTED_EDGE('',*,*,#10665,.F.);
#14314=ORIENTED_EDGE('',*,*,#10666,.T.);
#14315=ORIENTED_EDGE('',*,*,#10667,.T.);
#14316=ORIENTED_EDGE('',*,*,#10422,.F.);
#14317=ORIENTED_EDGE('',*,*,#10357,.T.);
#14318=ORIENTED_EDGE('',*,*,#10664,.T.);
#14319=ORIENTED_EDGE('',*,*,#10668,.T.);
#14320=ORIENTED_EDGE('',*,*,#10666,.F.);
#14321=ORIENTED_EDGE('',*,*,#10356,.T.);
#14322=ORIENTED_EDGE('',*,*,#10669,.T.);
#14323=ORIENTED_EDGE('',*,*,#10665,.T.);
#14324=ORIENTED_EDGE('',*,*,#10355,.T.);
#14325=ORIENTED_EDGE('',*,*,#10670,.T.);
#14326=ORIENTED_EDGE('',*,*,#10671,.F.);
#14327=ORIENTED_EDGE('',*,*,#10672,.F.);
#14328=ORIENTED_EDGE('',*,*,#10673,.F.);
#14329=ORIENTED_EDGE('',*,*,#10354,.T.);
#14330=ORIENTED_EDGE('',*,*,#10672,.T.);
#14331=ORIENTED_EDGE('',*,*,#10674,.T.);
#14332=ORIENTED_EDGE('',*,*,#10670,.F.);
#14333=ORIENTED_EDGE('',*,*,#10675,.T.);
#14334=ORIENTED_EDGE('',*,*,#10673,.T.);
#14335=ORIENTED_EDGE('',*,*,#10353,.T.);
#14336=ORIENTED_EDGE('',*,*,#10676,.T.);
#14337=ORIENTED_EDGE('',*,*,#10352,.T.);
#14338=ORIENTED_EDGE('',*,*,#10677,.T.);
#14339=ORIENTED_EDGE('',*,*,#10678,.T.);
#14340=ORIENTED_EDGE('',*,*,#10676,.F.);
#14341=ORIENTED_EDGE('',*,*,#10679,.F.);
#14342=ORIENTED_EDGE('',*,*,#10680,.F.);
#14343=ORIENTED_EDGE('',*,*,#10681,.F.);
#14344=ORIENTED_EDGE('',*,*,#10351,.T.);
#14345=ORIENTED_EDGE('',*,*,#10680,.T.);
#14346=ORIENTED_EDGE('',*,*,#10682,.T.);
#14347=ORIENTED_EDGE('',*,*,#10677,.F.);
#14348=ORIENTED_EDGE('',*,*,#10683,.F.);
#14349=ORIENTED_EDGE('',*,*,#10684,.F.);
#14350=ORIENTED_EDGE('',*,*,#10685,.F.);
#14351=ORIENTED_EDGE('',*,*,#10684,.T.);
#14352=ORIENTED_EDGE('',*,*,#10686,.T.);
#14353=ORIENTED_EDGE('',*,*,#10681,.T.);
#14354=ORIENTED_EDGE('',*,*,#10350,.T.);
#14355=ORIENTED_EDGE('',*,*,#10687,.F.);
#14356=ORIENTED_EDGE('',*,*,#10688,.F.);
#14357=ORIENTED_EDGE('',*,*,#10689,.F.);
#14358=ORIENTED_EDGE('',*,*,#10688,.T.);
#14359=ORIENTED_EDGE('',*,*,#10690,.T.);
#14360=ORIENTED_EDGE('',*,*,#10685,.T.);
#14361=ORIENTED_EDGE('',*,*,#10349,.T.);
#14362=ORIENTED_EDGE('',*,*,#10429,.F.);
#14363=ORIENTED_EDGE('',*,*,#10691,.T.);
#14364=ORIENTED_EDGE('',*,*,#10689,.T.);
#14365=ORIENTED_EDGE('',*,*,#10348,.T.);
#14366=ORIENTED_EDGE('',*,*,#10692,.T.);
#14367=ORIENTED_EDGE('',*,*,#10693,.T.);
#14368=ORIENTED_EDGE('',*,*,#10687,.T.);
#14369=ORIENTED_EDGE('',*,*,#10694,.T.);
#14370=ORIENTED_EDGE('',*,*,#10614,.F.);
#14371=ORIENTED_EDGE('',*,*,#10587,.T.);
#14372=ORIENTED_EDGE('',*,*,#10695,.T.);
#14373=ORIENTED_EDGE('',*,*,#10696,.T.);
#14374=ORIENTED_EDGE('',*,*,#10697,.T.);
#14375=ORIENTED_EDGE('',*,*,#10698,.T.);
#14376=ORIENTED_EDGE('',*,*,#10683,.T.);
#14377=ORIENTED_EDGE('',*,*,#10699,.T.);
#14378=ORIENTED_EDGE('',*,*,#10697,.F.);
#14379=ORIENTED_EDGE('',*,*,#10700,.T.);
#14380=ORIENTED_EDGE('',*,*,#10701,.T.);
#14381=ORIENTED_EDGE('',*,*,#10702,.T.);
#14382=ORIENTED_EDGE('',*,*,#10703,.T.);
#14383=ORIENTED_EDGE('',*,*,#10679,.T.);
#14384=ORIENTED_EDGE('',*,*,#10704,.T.);
#14385=ORIENTED_EDGE('',*,*,#10702,.F.);
#14386=ORIENTED_EDGE('',*,*,#10705,.T.);
#14387=ORIENTED_EDGE('',*,*,#10706,.T.);
#14388=ORIENTED_EDGE('',*,*,#10707,.T.);
#14389=ORIENTED_EDGE('',*,*,#10708,.T.);
#14390=ORIENTED_EDGE('',*,*,#10671,.T.);
#14391=ORIENTED_EDGE('',*,*,#10709,.T.);
#14392=ORIENTED_EDGE('',*,*,#10707,.F.);
#14393=ORIENTED_EDGE('',*,*,#10710,.T.);
#14394=ORIENTED_EDGE('',*,*,#10711,.T.);
#14395=ORIENTED_EDGE('',*,*,#10712,.T.);
#14396=ORIENTED_EDGE('',*,*,#10713,.T.);
#14397=ORIENTED_EDGE('',*,*,#10663,.T.);
#14398=ORIENTED_EDGE('',*,*,#10714,.T.);
#14399=ORIENTED_EDGE('',*,*,#10712,.F.);
#14400=ORIENTED_EDGE('',*,*,#10715,.T.);
#14401=ORIENTED_EDGE('',*,*,#10716,.T.);
#14402=ORIENTED_EDGE('',*,*,#10421,.F.);
#14403=ORIENTED_EDGE('',*,*,#10717,.T.);
#14404=ORIENTED_EDGE('',*,*,#10718,.T.);
#14405=ORIENTED_EDGE('',*,*,#10719,.T.);
#14406=ORIENTED_EDGE('',*,*,#10695,.F.);
#14407=ORIENTED_EDGE('',*,*,#10720,.T.);
#14408=ORIENTED_EDGE('',*,*,#10692,.F.);
#14409=ORIENTED_EDGE('',*,*,#10718,.F.);
#14410=ORIENTED_EDGE('',*,*,#10721,.T.);
#14411=ORIENTED_EDGE('',*,*,#10661,.F.);
#14412=ORIENTED_EDGE('',*,*,#10716,.F.);
#14413=ORIENTED_EDGE('',*,*,#10579,.T.);
#14414=ORIENTED_EDGE('',*,*,#10722,.F.);
#14415=ORIENTED_EDGE('',*,*,#10723,.T.);
#14416=ORIENTED_EDGE('',*,*,#10715,.F.);
#14417=ORIENTED_EDGE('',*,*,#10724,.T.);
#14418=ORIENTED_EDGE('',*,*,#10725,.F.);
#14419=ORIENTED_EDGE('',*,*,#10580,.T.);
#14420=ORIENTED_EDGE('',*,*,#10714,.F.);
#14421=ORIENTED_EDGE('',*,*,#10669,.F.);
#14422=ORIENTED_EDGE('',*,*,#10726,.T.);
#14423=ORIENTED_EDGE('',*,*,#10724,.F.);
#14424=ORIENTED_EDGE('',*,*,#10674,.F.);
#14425=ORIENTED_EDGE('',*,*,#10708,.F.);
#14426=ORIENTED_EDGE('',*,*,#10727,.F.);
#14427=ORIENTED_EDGE('',*,*,#10726,.F.);
#14428=ORIENTED_EDGE('',*,*,#10711,.F.);
#14429=ORIENTED_EDGE('',*,*,#10581,.T.);
#14430=ORIENTED_EDGE('',*,*,#10725,.T.);
#14431=ORIENTED_EDGE('',*,*,#10727,.T.);
#14432=ORIENTED_EDGE('',*,*,#10710,.F.);
#14433=ORIENTED_EDGE('',*,*,#10728,.T.);
#14434=ORIENTED_EDGE('',*,*,#10729,.F.);
#14435=ORIENTED_EDGE('',*,*,#10582,.T.);
#14436=ORIENTED_EDGE('',*,*,#10709,.F.);
#14437=ORIENTED_EDGE('',*,*,#10675,.F.);
#14438=ORIENTED_EDGE('',*,*,#10730,.T.);
#14439=ORIENTED_EDGE('',*,*,#10728,.F.);
#14440=ORIENTED_EDGE('',*,*,#10678,.F.);
#14441=ORIENTED_EDGE('',*,*,#10731,.T.);
#14442=ORIENTED_EDGE('',*,*,#10732,.F.);
#14443=ORIENTED_EDGE('',*,*,#10730,.F.);
#14444=ORIENTED_EDGE('',*,*,#10682,.F.);
#14445=ORIENTED_EDGE('',*,*,#10703,.F.);
#14446=ORIENTED_EDGE('',*,*,#10733,.F.);
#14447=ORIENTED_EDGE('',*,*,#10731,.F.);
#14448=ORIENTED_EDGE('',*,*,#10706,.F.);
#14449=ORIENTED_EDGE('',*,*,#10584,.T.);
#14450=ORIENTED_EDGE('',*,*,#10734,.T.);
#14451=ORIENTED_EDGE('',*,*,#10733,.T.);
#14452=ORIENTED_EDGE('',*,*,#10704,.F.);
#14453=ORIENTED_EDGE('',*,*,#10686,.F.);
#14454=ORIENTED_EDGE('',*,*,#10698,.F.);
#14455=ORIENTED_EDGE('',*,*,#10735,.F.);
#14456=ORIENTED_EDGE('',*,*,#10705,.F.);
#14457=ORIENTED_EDGE('',*,*,#10735,.T.);
#14458=ORIENTED_EDGE('',*,*,#10701,.F.);
#14459=ORIENTED_EDGE('',*,*,#10585,.T.);
#14460=ORIENTED_EDGE('',*,*,#10699,.F.);
#14461=ORIENTED_EDGE('',*,*,#10690,.F.);
#14462=ORIENTED_EDGE('',*,*,#10693,.F.);
#14463=ORIENTED_EDGE('',*,*,#10736,.F.);
#14464=ORIENTED_EDGE('',*,*,#10700,.F.);
#14465=ORIENTED_EDGE('',*,*,#10736,.T.);
#14466=ORIENTED_EDGE('',*,*,#10720,.F.);
#14467=ORIENTED_EDGE('',*,*,#10586,.T.);
#14468=ORIENTED_EDGE('',*,*,#10691,.F.);
#14469=ORIENTED_EDGE('',*,*,#10618,.F.);
#14470=ORIENTED_EDGE('',*,*,#10696,.F.);
#14471=ORIENTED_EDGE('',*,*,#10694,.F.);
#14472=ORIENTED_EDGE('',*,*,#10583,.T.);
#14473=ORIENTED_EDGE('',*,*,#10729,.T.);
#14474=ORIENTED_EDGE('',*,*,#10732,.T.);
#14475=ORIENTED_EDGE('',*,*,#10734,.F.);
#14476=ORIENTED_EDGE('',*,*,#10721,.F.);
#14477=ORIENTED_EDGE('',*,*,#10737,.T.);
#14478=ORIENTED_EDGE('',*,*,#10738,.T.);
#14479=ORIENTED_EDGE('',*,*,#10577,.T.);
#14480=ORIENTED_EDGE('',*,*,#10722,.T.);
#14481=ORIENTED_EDGE('',*,*,#10578,.T.);
#14482=ORIENTED_EDGE('',*,*,#10738,.F.);
#14483=ORIENTED_EDGE('',*,*,#10739,.T.);
#14484=ORIENTED_EDGE('',*,*,#10713,.F.);
#14485=ORIENTED_EDGE('',*,*,#10723,.F.);
#14486=ORIENTED_EDGE('',*,*,#10740,.F.);
#14487=ORIENTED_EDGE('',*,*,#10668,.F.);
#14488=ORIENTED_EDGE('',*,*,#10667,.F.);
#14489=ORIENTED_EDGE('',*,*,#10740,.T.);
#14490=ORIENTED_EDGE('',*,*,#10739,.F.);
#14491=ORIENTED_EDGE('',*,*,#10741,.F.);
#14492=ORIENTED_EDGE('',*,*,#10423,.F.);
#14493=ORIENTED_EDGE('',*,*,#10741,.T.);
#14494=ORIENTED_EDGE('',*,*,#10737,.F.);
#14495=ORIENTED_EDGE('',*,*,#10717,.F.);
#14496=ORIENTED_EDGE('',*,*,#10651,.F.);
#14497=ORIENTED_EDGE('',*,*,#10660,.T.);
#14498=ORIENTED_EDGE('',*,*,#10659,.F.);
#14499=ORIENTED_EDGE('',*,*,#10595,.T.);
#14500=ORIENTED_EDGE('',*,*,#10632,.F.);
#14501=ORIENTED_EDGE('',*,*,#10742,.T.);
#14502=ORIENTED_EDGE('',*,*,#10652,.F.);
#14503=ORIENTED_EDGE('',*,*,#10594,.T.);
#14504=ORIENTED_EDGE('',*,*,#10633,.F.);
#14505=ORIENTED_EDGE('',*,*,#10593,.T.);
#14506=ORIENTED_EDGE('',*,*,#10635,.F.);
#14507=ORIENTED_EDGE('',*,*,#10743,.T.);
#14508=ORIENTED_EDGE('',*,*,#10628,.F.);
#14509=ORIENTED_EDGE('',*,*,#10654,.F.);
#14510=ORIENTED_EDGE('',*,*,#10742,.F.);
#14511=ORIENTED_EDGE('',*,*,#10631,.F.);
#14512=ORIENTED_EDGE('',*,*,#10630,.F.);
#14513=ORIENTED_EDGE('',*,*,#10743,.F.);
#14514=ORIENTED_EDGE('',*,*,#10638,.F.);
#14515=ORIENTED_EDGE('',*,*,#10624,.F.);
#14516=ORIENTED_EDGE('',*,*,#10604,.T.);
#14517=ORIENTED_EDGE('',*,*,#10744,.T.);
#14518=ORIENTED_EDGE('',*,*,#10383,.T.);
#14519=ORIENTED_EDGE('',*,*,#10384,.T.);
#14520=ORIENTED_EDGE('',*,*,#10744,.F.);
#14521=ORIENTED_EDGE('',*,*,#10745,.T.);
#14522=ORIENTED_EDGE('',*,*,#10404,.T.);
#14523=ORIENTED_EDGE('',*,*,#10746,.T.);
#14524=ORIENTED_EDGE('',*,*,#10597,.T.);
#14525=ORIENTED_EDGE('',*,*,#10747,.T.);
#14526=ORIENTED_EDGE('',*,*,#10598,.T.);
#14527=ORIENTED_EDGE('',*,*,#10746,.F.);
#14528=ORIENTED_EDGE('',*,*,#10748,.T.);
#14529=ORIENTED_EDGE('',*,*,#10749,.T.);
#14530=ORIENTED_EDGE('',*,*,#10599,.T.);
#14531=ORIENTED_EDGE('',*,*,#10747,.F.);
#14532=ORIENTED_EDGE('',*,*,#10750,.T.);
#14533=ORIENTED_EDGE('',*,*,#10745,.F.);
#14534=ORIENTED_EDGE('',*,*,#10600,.T.);
#14535=ORIENTED_EDGE('',*,*,#10749,.F.);
#14536=ORIENTED_EDGE('',*,*,#10401,.T.);
#14537=ORIENTED_EDGE('',*,*,#10399,.F.);
#14538=ORIENTED_EDGE('',*,*,#10751,.T.);
#14539=ORIENTED_EDGE('',*,*,#10748,.F.);
#14540=ORIENTED_EDGE('',*,*,#10403,.F.);
#14541=ORIENTED_EDGE('',*,*,#10253,.T.);
#14542=ORIENTED_EDGE('',*,*,#10254,.T.);
#14543=ORIENTED_EDGE('',*,*,#10752,.T.);
#14544=ORIENTED_EDGE('',*,*,#10603,.T.);
#14545=ORIENTED_EDGE('',*,*,#10752,.F.);
#14546=ORIENTED_EDGE('',*,*,#10753,.T.);
#14547=ORIENTED_EDGE('',*,*,#10754,.T.);
#14548=ORIENTED_EDGE('',*,*,#10601,.T.);
#14549=ORIENTED_EDGE('',*,*,#10754,.F.);
#14550=ORIENTED_EDGE('',*,*,#10755,.T.);
#14551=ORIENTED_EDGE('',*,*,#10756,.F.);
#14552=ORIENTED_EDGE('',*,*,#10757,.F.);
#14553=ORIENTED_EDGE('',*,*,#10758,.T.);
#14554=ORIENTED_EDGE('',*,*,#10755,.F.);
#14555=ORIENTED_EDGE('',*,*,#10753,.F.);
#14556=ORIENTED_EDGE('',*,*,#10758,.F.);
#14557=ORIENTED_EDGE('',*,*,#10756,.T.);
#14558=ORIENTED_EDGE('',*,*,#10757,.T.);
#14559=ORIENTED_EDGE('',*,*,#10759,.T.);
#14560=ORIENTED_EDGE('',*,*,#10389,.T.);
#14561=ORIENTED_EDGE('',*,*,#10390,.T.);
#14562=ORIENTED_EDGE('',*,*,#10759,.F.);
#14563=ORIENTED_EDGE('',*,*,#10398,.F.);
#14564=ORIENTED_EDGE('',*,*,#10402,.T.);
#14565=ORIENTED_EDGE('',*,*,#10750,.F.);
#14566=ORIENTED_EDGE('',*,*,#10751,.F.);
#14567=ORIENTED_EDGE('',*,*,#10419,.F.);
#14568=ORIENTED_EDGE('',*,*,#10719,.F.);
#14569=ORIENTED_EDGE('',*,*,#10662,.F.);
#14570=ORIENTED_EDGE('',*,*,#10573,.F.);
#19047=ADVANCED_FACE('',(#5113),#1183,.T.);
#19048=ADVANCED_FACE('',(#5114),#4558,.F.);
#19049=ADVANCED_FACE('',(#5115),#227,.F.);
#19050=ADVANCED_FACE('',(#5116),#4559,.T.);
#19051=ADVANCED_FACE('',(#5117),#117,.T.);
#19052=ADVANCED_FACE('',(#5118),#118,.T.);
#19053=ADVANCED_FACE('',(#5119),#4560,.T.);
#19054=ADVANCED_FACE('',(#5120),#1184,.T.);
#19055=ADVANCED_FACE('',(#5121),#4561,.F.);
#19056=ADVANCED_FACE('',(#5122),#4562,.T.);
#19057=ADVANCED_FACE('',(#5123),#119,.T.);
#19058=ADVANCED_FACE('',(#5124),#120,.T.);
#19059=ADVANCED_FACE('',(#5125),#1185,.T.);
#19060=ADVANCED_FACE('',(#5126),#1364,.F.);
#19061=ADVANCED_FACE('',(#5127),#4563,.T.);
#19062=ADVANCED_FACE('',(#5128),#121,.T.);
#19063=ADVANCED_FACE('',(#5129),#122,.T.);
#19064=ADVANCED_FACE('',(#5130),#4564,.T.);
#19065=ADVANCED_FACE('',(#5131),#4565,.F.);
#19066=ADVANCED_FACE('',(#5132),#4566,.T.);
#19067=ADVANCED_FACE('',(#5133),#123,.T.);
#19068=ADVANCED_FACE('',(#5134),#124,.T.);
#19069=ADVANCED_FACE('',(#5135),#1186,.T.);
#19070=ADVANCED_FACE('',(#5136),#1365,.F.);
#19071=ADVANCED_FACE('',(#5137),#4567,.T.);
#19072=ADVANCED_FACE('',(#5138),#125,.T.);
#19073=ADVANCED_FACE('',(#5139),#126,.T.);
#19074=ADVANCED_FACE('',(#5140),#1187,.T.);
#19075=ADVANCED_FACE('',(#5141),#4568,.T.);
#19076=ADVANCED_FACE('',(#5142),#1366,.F.);
#19077=ADVANCED_FACE('',(#5143),#4569,.T.);
#19078=ADVANCED_FACE('',(#5144),#127,.T.);
#19079=ADVANCED_FACE('',(#5145),#128,.T.);
#19080=ADVANCED_FACE('',(#5146),#4570,.T.);
#19081=ADVANCED_FACE('',(#5147),#4571,.F.);
#19082=ADVANCED_FACE('',(#5148),#1188,.T.);
#19083=ADVANCED_FACE('',(#5149,#1703,#1704,#1705,#1706,#1707,#1708,#1709),
#1367,.F.);
#19084=ADVANCED_FACE('',(#5150),#4572,.F.);
#19085=ADVANCED_FACE('',(#5151),#1189,.T.);
#19086=ADVANCED_FACE('',(#5152),#4573,.F.);
#19087=ADVANCED_FACE('',(#5153),#1190,.T.);
#19088=ADVANCED_FACE('',(#5154),#4574,.T.);
#19089=ADVANCED_FACE('',(#5155),#1191,.T.);
#19090=ADVANCED_FACE('',(#5156),#4575,.T.);
#19091=ADVANCED_FACE('',(#5157),#1192,.T.);
#19092=ADVANCED_FACE('',(#5158),#4576,.F.);
#19093=ADVANCED_FACE('',(#5159),#1368,.F.);
#19094=ADVANCED_FACE('',(#5160),#4577,.T.);
#19095=ADVANCED_FACE('',(#5161),#1193,.T.);
#19096=ADVANCED_FACE('',(#5162),#129,.T.);
#19097=ADVANCED_FACE('',(#5163),#4578,.T.);
#19098=ADVANCED_FACE('',(#5164),#130,.T.);
#19099=ADVANCED_FACE('',(#5165),#1369,.F.);
#19100=ADVANCED_FACE('',(#5166),#4579,.T.);
#19101=ADVANCED_FACE('',(#5167),#1194,.T.);
#19102=ADVANCED_FACE('',(#5168),#4580,.T.);
#19103=ADVANCED_FACE('',(#5169),#131,.T.);
#19104=ADVANCED_FACE('',(#5170),#4581,.T.);
#19105=ADVANCED_FACE('',(#5171),#132,.T.);
#19106=ADVANCED_FACE('',(#5172),#133,.T.);
#19107=ADVANCED_FACE('',(#5173),#4582,.T.);
#19108=ADVANCED_FACE('',(#5174),#134,.T.);
#19109=ADVANCED_FACE('',(#5175),#4583,.T.);
#19110=ADVANCED_FACE('',(#5176),#135,.T.);
#19111=ADVANCED_FACE('',(#5177),#4584,.T.);
#19112=ADVANCED_FACE('',(#5178),#4585,.T.);
#19113=ADVANCED_FACE('',(#5179),#136,.T.);
#19114=ADVANCED_FACE('',(#5180),#4586,.T.);
#19115=ADVANCED_FACE('',(#5181),#137,.T.);
#19116=ADVANCED_FACE('',(#5182),#4587,.T.);
#19117=ADVANCED_FACE('',(#5183),#138,.T.);
#19118=ADVANCED_FACE('',(#5184),#4588,.T.);
#19119=ADVANCED_FACE('',(#5185),#139,.T.);
#19120=ADVANCED_FACE('',(#5186),#1370,.T.);
#19121=ADVANCED_FACE('',(#5187),#1371,.T.);
#19122=ADVANCED_FACE('',(#5188),#4589,.T.);
#19123=ADVANCED_FACE('',(#5189),#4590,.T.);
#19124=ADVANCED_FACE('',(#5190),#1372,.T.);
#19125=ADVANCED_FACE('',(#5191),#140,.T.);
#19126=ADVANCED_FACE('',(#5192),#141,.T.);
#19127=ADVANCED_FACE('',(#5193),#4591,.T.);
#19128=ADVANCED_FACE('',(#5194),#1195,.T.);
#19129=ADVANCED_FACE('',(#5195),#142,.T.);
#19130=ADVANCED_FACE('',(#5196),#4592,.T.);
#19131=ADVANCED_FACE('',(#5197),#1196,.T.);
#19132=ADVANCED_FACE('',(#5198),#4593,.T.);
#19133=ADVANCED_FACE('',(#5199),#1197,.T.);
#19134=ADVANCED_FACE('',(#5200),#4594,.T.);
#19135=ADVANCED_FACE('',(#5201),#143,.T.);
#19136=ADVANCED_FACE('',(#5202),#1198,.T.);
#19137=ADVANCED_FACE('',(#5203),#144,.T.);
#19138=ADVANCED_FACE('',(#5204),#1199,.T.);
#19139=ADVANCED_FACE('',(#5205),#4595,.T.);
#19140=ADVANCED_FACE('',(#5206),#1373,.F.);
#19141=ADVANCED_FACE('',(#5207),#4596,.T.);
#19142=ADVANCED_FACE('',(#5208),#4597,.F.);
#19143=ADVANCED_FACE('',(#5209),#4598,.T.);
#19144=ADVANCED_FACE('',(#5210),#1200,.T.);
#19145=ADVANCED_FACE('',(#5211),#4599,.F.);
#19146=ADVANCED_FACE('',(#5212),#145,.T.);
#19147=ADVANCED_FACE('',(#5213),#4600,.T.);
#19148=ADVANCED_FACE('',(#5214),#146,.T.);
#19149=ADVANCED_FACE('',(#5215),#4601,.T.);
#19150=ADVANCED_FACE('',(#5216),#147,.T.);
#19151=ADVANCED_FACE('',(#5217),#4602,.T.);
#19152=ADVANCED_FACE('',(#5218),#148,.T.);
#19153=ADVANCED_FACE('',(#5219),#4603,.T.);
#19154=ADVANCED_FACE('',(#5220),#4604,.T.);
#19155=ADVANCED_FACE('',(#5221),#4605,.T.);
#19156=ADVANCED_FACE('',(#5222),#149,.T.);
#19157=ADVANCED_FACE('',(#5223),#4606,.T.);
#19158=ADVANCED_FACE('',(#5224),#4607,.T.);
#19159=ADVANCED_FACE('',(#5225),#4608,.T.);
#19160=ADVANCED_FACE('',(#5226),#150,.T.);
#19161=ADVANCED_FACE('',(#5227),#4609,.T.);
#19162=ADVANCED_FACE('',(#5228),#151,.T.);
#19163=ADVANCED_FACE('',(#5229),#4610,.T.);
#19164=ADVANCED_FACE('',(#5230),#152,.T.);
#19165=ADVANCED_FACE('',(#5231),#4611,.T.);
#19166=ADVANCED_FACE('',(#5232),#153,.T.);
#19167=ADVANCED_FACE('',(#5233),#4612,.T.);
#19168=ADVANCED_FACE('',(#5234),#154,.T.);
#19169=ADVANCED_FACE('',(#5235),#4613,.T.);
#19170=ADVANCED_FACE('',(#5236),#155,.T.);
#19171=ADVANCED_FACE('',(#5237),#1374,.T.);
#19172=ADVANCED_FACE('',(#5238),#4614,.T.);
#19173=ADVANCED_FACE('',(#5239),#4615,.T.);
#19174=ADVANCED_FACE('',(#5240),#1375,.T.);
#19175=ADVANCED_FACE('',(#5241),#4616,.T.);
#19176=ADVANCED_FACE('',(#5242),#4617,.T.);
#19177=ADVANCED_FACE('',(#5243),#1376,.T.);
#19178=ADVANCED_FACE('',(#5244),#1377,.T.);
#19179=ADVANCED_FACE('',(#5245),#1378,.T.);
#19180=ADVANCED_FACE('',(#5246),#4618,.T.);
#19181=ADVANCED_FACE('',(#5247),#4619,.T.);
#19182=ADVANCED_FACE('',(#5248),#1379,.T.);
#19183=ADVANCED_FACE('',(#5249),#1201,.T.);
#19184=ADVANCED_FACE('',(#5250,#1710,#1711,#1712,#1713,#1714,#1715,#1716),
#1380,.T.);
#19185=ADVANCED_FACE('',(#5251),#156,.T.);
#19186=ADVANCED_FACE('',(#5252),#4620,.T.);
#19187=ADVANCED_FACE('',(#5253),#4621,.T.);
#19188=ADVANCED_FACE('',(#5254),#4622,.T.);
#19189=ADVANCED_FACE('',(#5255),#157,.T.);
#19190=ADVANCED_FACE('',(#5256),#158,.T.);
#19191=ADVANCED_FACE('',(#5257),#4623,.F.);
#19192=ADVANCED_FACE('',(#5258),#1381,.F.);
#19193=ADVANCED_FACE('',(#5259),#4624,.T.);
#19194=ADVANCED_FACE('',(#5260),#4625,.T.);
#19195=ADVANCED_FACE('',(#5261),#4626,.T.);
#19196=ADVANCED_FACE('',(#5262),#159,.T.);
#19197=ADVANCED_FACE('',(#5263),#4627,.T.);
#19198=ADVANCED_FACE('',(#5264),#1382,.T.);
#19199=ADVANCED_FACE('',(#5265),#1383,.T.);
#19200=ADVANCED_FACE('',(#5266),#1384,.T.);
#19201=ADVANCED_FACE('',(#5267),#4628,.T.);
#19202=ADVANCED_FACE('',(#5268),#160,.T.);
#19203=ADVANCED_FACE('',(#5269),#161,.T.);
#19204=ADVANCED_FACE('',(#5270),#4629,.T.);
#19205=ADVANCED_FACE('',(#5271),#162,.T.);
#19206=ADVANCED_FACE('',(#5272),#1202,.T.);
#19207=ADVANCED_FACE('',(#5273),#4630,.T.);
#19208=ADVANCED_FACE('',(#5274),#163,.T.);
#19209=ADVANCED_FACE('',(#5275),#164,.T.);
#19210=ADVANCED_FACE('',(#5276),#4631,.T.);
#19211=ADVANCED_FACE('',(#5277),#165,.T.);
#19212=ADVANCED_FACE('',(#5278),#4632,.F.);
#19213=ADVANCED_FACE('',(#5279),#1203,.T.);
#19214=ADVANCED_FACE('',(#5280),#166,.T.);
#19215=ADVANCED_FACE('',(#5281),#4633,.T.);
#19216=ADVANCED_FACE('',(#5282),#1204,.T.);
#19217=ADVANCED_FACE('',(#5283),#167,.T.);
#19218=ADVANCED_FACE('',(#5284),#1205,.T.);
#19219=ADVANCED_FACE('',(#5285),#168,.T.);
#19220=ADVANCED_FACE('',(#5286),#4634,.T.);
#19221=ADVANCED_FACE('',(#5287),#4635,.T.);
#19222=ADVANCED_FACE('',(#5288),#4636,.T.);
#19223=ADVANCED_FACE('',(#5289),#169,.T.);
#19224=ADVANCED_FACE('',(#5290),#1385,.F.);
#19225=ADVANCED_FACE('',(#5291),#4637,.F.);
#19226=ADVANCED_FACE('',(#5292),#4638,.T.);
#19227=ADVANCED_FACE('',(#5293),#170,.T.);
#19228=ADVANCED_FACE('',(#5294),#1206,.T.);
#19229=ADVANCED_FACE('',(#5295),#4639,.T.);
#19230=ADVANCED_FACE('',(#5296),#4640,.T.);
#19231=ADVANCED_FACE('',(#5297),#171,.T.);
#19232=ADVANCED_FACE('',(#5298),#4641,.T.);
#19233=ADVANCED_FACE('',(#5299),#4642,.T.);
#19234=ADVANCED_FACE('',(#5300),#4643,.T.);
#19235=ADVANCED_FACE('',(#5301),#172,.T.);
#19236=ADVANCED_FACE('',(#5302),#4644,.T.);
#19237=ADVANCED_FACE('',(#5303),#173,.T.);
#19238=ADVANCED_FACE('',(#5304),#4645,.T.);
#19239=ADVANCED_FACE('',(#5305),#174,.T.);
#19240=ADVANCED_FACE('',(#5306),#4646,.T.);
#19241=ADVANCED_FACE('',(#5307),#4647,.T.);
#19242=ADVANCED_FACE('',(#5308),#4648,.T.);
#19243=ADVANCED_FACE('',(#5309),#4649,.T.);
#19244=ADVANCED_FACE('',(#5310),#4650,.T.);
#19245=ADVANCED_FACE('',(#5311),#175,.T.);
#19246=ADVANCED_FACE('',(#5312),#4651,.T.);
#19247=ADVANCED_FACE('',(#5313),#176,.T.);
#19248=ADVANCED_FACE('',(#5314),#4652,.T.);
#19249=ADVANCED_FACE('',(#5315),#177,.T.);
#19250=ADVANCED_FACE('',(#5316),#4653,.T.);
#19251=ADVANCED_FACE('',(#5317),#178,.T.);
#19252=ADVANCED_FACE('',(#5318),#4654,.T.);
#19253=ADVANCED_FACE('',(#5319),#179,.T.);
#19254=ADVANCED_FACE('',(#5320),#180,.T.);
#19255=ADVANCED_FACE('',(#5321),#4655,.T.);
#19256=ADVANCED_FACE('',(#5322),#4656,.T.);
#19257=ADVANCED_FACE('',(#5323),#1386,.T.);
#19258=ADVANCED_FACE('',(#5324),#1387,.T.);
#19259=ADVANCED_FACE('',(#5325),#4657,.T.);
#19260=ADVANCED_FACE('',(#5326),#4658,.T.);
#19261=ADVANCED_FACE('',(#5327),#1388,.T.);
#19262=ADVANCED_FACE('',(#5328),#1389,.T.);
#19263=ADVANCED_FACE('',(#5329),#1390,.T.);
#19264=ADVANCED_FACE('',(#5330),#4659,.T.);
#19265=ADVANCED_FACE('',(#5331),#1391,.T.);
#19266=ADVANCED_FACE('',(#5332),#4660,.T.);
#19267=ADVANCED_FACE('',(#5333),#1392,.T.);
#19268=ADVANCED_FACE('',(#5334),#4661,.T.);
#19269=ADVANCED_FACE('',(#5335),#1393,.T.);
#19270=ADVANCED_FACE('',(#5336),#4662,.T.);
#19271=ADVANCED_FACE('',(#5337),#4663,.T.);
#19272=ADVANCED_FACE('',(#5338),#1207,.T.);
#19273=ADVANCED_FACE('',(#5339),#1394,.T.);
#19274=ADVANCED_FACE('',(#5340),#4664,.F.);
#19275=ADVANCED_FACE('',(#5341),#1395,.T.);
#19276=ADVANCED_FACE('',(#5342),#4665,.T.);
#19277=ADVANCED_FACE('',(#5343),#1208,.T.);
#19278=ADVANCED_FACE('',(#5344),#4666,.T.);
#19279=ADVANCED_FACE('',(#5345),#4667,.F.);
#19280=ADVANCED_FACE('',(#5346),#1396,.F.);
#19281=ADVANCED_FACE('',(#5347),#1209,.T.);
#19282=ADVANCED_FACE('',(#5348),#4668,.T.);
#19283=ADVANCED_FACE('',(#5349),#1210,.T.);
#19284=ADVANCED_FACE('',(#5350),#4669,.T.);
#19285=ADVANCED_FACE('',(#5351),#1211,.T.);
#19286=ADVANCED_FACE('',(#5352),#4670,.F.);
#19287=ADVANCED_FACE('',(#5353),#1212,.T.);
#19288=ADVANCED_FACE('',(#5354),#1213,.T.);
#19289=ADVANCED_FACE('',(#5355),#228,.F.);
#19290=ADVANCED_FACE('',(#5356),#1214,.T.);
#19291=ADVANCED_FACE('',(#5357),#1397,.F.);
#19292=ADVANCED_FACE('',(#5358),#1398,.T.);
#20118=CLOSED_SHELL('',(#19047,#19048,#19049,#19050,#19051,#19052,#19053,
#19054,#19055,#19056,#19057,#19058,#19059,#19060,#19061,#19062,#19063,#19064,
#19065,#19066,#19067,#19068,#19069,#19070,#19071,#19072,#19073,#19074,#19075,
#19076,#19077,#19078,#19079,#19080,#19081,#19082,#19083,#19084,#19085,#19086,
#19087,#19088,#19089,#19090,#19091,#19092,#19093,#19094,#19095,#19096,#19097,
#19098,#19099,#19100,#19101,#19102,#19103,#19104,#19105,#19106,#19107,#19108,
#19109,#19110,#19111,#19112,#19113,#19114,#19115,#19116,#19117,#19118,#19119,
#19120,#19121,#19122,#19123,#19124,#19125,#19126,#19127,#19128,#19129,#19130,
#19131,#19132,#19133,#19134,#19135,#19136,#19137,#19138,#19139,#19140,#19141,
#19142,#19143,#19144,#19145,#19146,#19147,#19148,#19149,#19150,#19151,#19152,
#19153,#19154,#19155,#19156,#19157,#19158,#19159,#19160,#19161,#19162,#19163,
#19164,#19165,#19166,#19167,#19168,#19169,#19170,#19171,#19172,#19173,#19174,
#19175,#19176,#19177,#19178,#19179,#19180,#19181,#19182,#19183,#19184,#19185,
#19186,#19187,#19188,#19189,#19190,#19191,#19192,#19193,#19194,#19195,#19196,
#19197,#19198,#19199,#19200,#19201,#19202,#19203,#19204,#19205,#19206,#19207,
#19208,#19209,#19210,#19211,#19212,#19213,#19214,#19215,#19216,#19217,#19218,
#19219,#19220,#19221,#19222,#19223,#19224,#19225,#19226,#19227,#19228,#19229,
#19230,#19231,#19232,#19233,#19234,#19235,#19236,#19237,#19238,#19239,#19240,
#19241,#19242,#19243,#19244,#19245,#19246,#19247,#19248,#19249,#19250,#19251,
#19252,#19253,#19254,#19255,#19256,#19257,#19258,#19259,#19260,#19261,#19262,
#19263,#19264,#19265,#19266,#19267,#19268,#19269,#19270,#19271,#19272,#19273,
#19274,#19275,#19276,#19277,#19278,#19279,#19280,#19281,#19282,#19283,#19284,
#19285,#19286,#19287,#19288,#19289,#19290,#19291,#19292));
#20343=AXIS2_PLACEMENT_3D('',#59065,#22633,#22634);
#20344=AXIS2_PLACEMENT_3D('',#59066,#22635,#22636);
#20345=AXIS2_PLACEMENT_3D('',#59069,#22637,#22638);
#20346=AXIS2_PLACEMENT_3D('',#59071,#22639,#22640);
#20347=AXIS2_PLACEMENT_3D('',#59073,#22641,#22642);
#20348=AXIS2_PLACEMENT_3D('',#59074,#22643,#22644);
#20349=AXIS2_PLACEMENT_3D('',#59075,#22645,#22646);
#20350=AXIS2_PLACEMENT_3D('',#59076,#22647,#22648);
#20351=AXIS2_PLACEMENT_3D('',#59079,#22649,#22650);
#20352=AXIS2_PLACEMENT_3D('',#59080,#22651,#22652);
#20353=AXIS2_PLACEMENT_3D('',#59082,#22654,#22655);
#20354=AXIS2_PLACEMENT_3D('',#59086,#22657,#22658);
#20355=AXIS2_PLACEMENT_3D('',#59087,#22659,#22660);
#20356=AXIS2_PLACEMENT_3D('',#59088,#22661,#22662);
#20357=AXIS2_PLACEMENT_3D('',#59091,#22663,#22664);
#20358=AXIS2_PLACEMENT_3D('',#59095,#22666,#22667);
#20359=AXIS2_PLACEMENT_3D('',#59097,#22669,#22670);
#20360=AXIS2_PLACEMENT_3D('',#59099,#22671,#22672);
#20361=AXIS2_PLACEMENT_3D('',#59100,#22673,#22674);
#20362=AXIS2_PLACEMENT_3D('',#59101,#22675,#22676);
#20363=AXIS2_PLACEMENT_3D('',#59103,#22677,#22678);
#20364=AXIS2_PLACEMENT_3D('',#59104,#22679,#22680);
#20365=AXIS2_PLACEMENT_3D('',#59105,#22681,#22682);
#20366=AXIS2_PLACEMENT_3D('',#59109,#22684,#22685);
#20367=AXIS2_PLACEMENT_3D('',#59111,#22687,#22688);
#20368=AXIS2_PLACEMENT_3D('',#59113,#22689,#22690);
#20369=AXIS2_PLACEMENT_3D('',#59115,#22691,#22692);
#20370=AXIS2_PLACEMENT_3D('',#59116,#22693,#22694);
#20371=AXIS2_PLACEMENT_3D('',#59117,#22695,#22696);
#20372=AXIS2_PLACEMENT_3D('',#59119,#22697,#22698);
#20373=AXIS2_PLACEMENT_3D('',#59121,#22700,#22701);
#20374=AXIS2_PLACEMENT_3D('',#59123,#22702,#22703);
#20375=AXIS2_PLACEMENT_3D('',#59127,#22705,#22706);
#20376=AXIS2_PLACEMENT_3D('',#59129,#22708,#22709);
#20377=AXIS2_PLACEMENT_3D('',#59131,#22710,#22711);
#20378=AXIS2_PLACEMENT_3D('',#59132,#22712,#22713);
#20379=AXIS2_PLACEMENT_3D('',#59133,#22714,#22715);
#20380=AXIS2_PLACEMENT_3D('',#59134,#22716,#22717);
#20381=AXIS2_PLACEMENT_3D('',#59135,#22718,#22719);
#20382=AXIS2_PLACEMENT_3D('',#59137,#22720,#22721);
#20383=AXIS2_PLACEMENT_3D('',#59139,#22722,#22723);
#20384=AXIS2_PLACEMENT_3D('',#59140,#22724,#22725);
#20385=AXIS2_PLACEMENT_3D('',#59141,#22726,#22727);
#20386=AXIS2_PLACEMENT_3D('',#59143,#22729,#22730);
#20387=AXIS2_PLACEMENT_3D('',#59146,#22731,#22732);
#20388=AXIS2_PLACEMENT_3D('',#59149,#22734,#22735);
#20389=AXIS2_PLACEMENT_3D('',#59151,#22737,#22738);
#20390=AXIS2_PLACEMENT_3D('',#59152,#22739,#22740);
#20391=AXIS2_PLACEMENT_3D('',#59153,#22741,#22742);
#20392=AXIS2_PLACEMENT_3D('',#59155,#22743,#22744);
#20393=AXIS2_PLACEMENT_3D('',#59156,#22745,#22746);
#20394=AXIS2_PLACEMENT_3D('',#59157,#22747,#22748);
#20395=AXIS2_PLACEMENT_3D('',#59161,#22750,#22751);
#20396=AXIS2_PLACEMENT_3D('',#59163,#22753,#22754);
#20397=AXIS2_PLACEMENT_3D('',#59164,#22755,#22756);
#20398=AXIS2_PLACEMENT_3D('',#59165,#22757,#22758);
#20399=AXIS2_PLACEMENT_3D('',#59167,#22759,#22760);
#20400=AXIS2_PLACEMENT_3D('',#59171,#22762,#22763);
#20401=AXIS2_PLACEMENT_3D('',#59173,#22765,#22766);
#20402=AXIS2_PLACEMENT_3D('',#59175,#22767,#22768);
#20403=AXIS2_PLACEMENT_3D('',#59176,#22769,#22770);
#20404=AXIS2_PLACEMENT_3D('',#59177,#22771,#22772);
#20405=AXIS2_PLACEMENT_3D('',#59178,#22773,#22774);
#20406=AXIS2_PLACEMENT_3D('',#59179,#22775,#22776);
#20407=AXIS2_PLACEMENT_3D('',#59181,#22777,#22778);
#20408=AXIS2_PLACEMENT_3D('',#59183,#22779,#22780);
#20409=AXIS2_PLACEMENT_3D('',#59184,#22781,#22782);
#20410=AXIS2_PLACEMENT_3D('',#59185,#22783,#22784);
#20411=AXIS2_PLACEMENT_3D('',#59187,#22786,#22787);
#20412=AXIS2_PLACEMENT_3D('',#59190,#22788,#22789);
#20413=AXIS2_PLACEMENT_3D('',#59194,#22791,#22792);
#20414=AXIS2_PLACEMENT_3D('',#59196,#22794,#22795);
#20415=AXIS2_PLACEMENT_3D('',#59198,#22796,#22797);
#20416=AXIS2_PLACEMENT_3D('',#59199,#22798,#22799);
#20417=AXIS2_PLACEMENT_3D('',#59200,#22800,#22801);
#20418=AXIS2_PLACEMENT_3D('',#59202,#22802,#22803);
#20419=AXIS2_PLACEMENT_3D('',#59203,#22804,#22805);
#20420=AXIS2_PLACEMENT_3D('',#59204,#22806,#22807);
#20421=AXIS2_PLACEMENT_3D('',#59206,#22808,#22809);
#20422=AXIS2_PLACEMENT_3D('',#59208,#22810,#22811);
#20423=AXIS2_PLACEMENT_3D('',#59209,#22812,#22813);
#20424=AXIS2_PLACEMENT_3D('',#59210,#22814,#22815);
#20425=AXIS2_PLACEMENT_3D('',#59214,#22817,#22818);
#20426=AXIS2_PLACEMENT_3D('',#59216,#22820,#22821);
#20427=AXIS2_PLACEMENT_3D('',#59220,#22824,#22825);
#20428=AXIS2_PLACEMENT_3D('',#59223,#22826,#22827);
#20429=AXIS2_PLACEMENT_3D('',#59226,#22829,#22830);
#20430=AXIS2_PLACEMENT_3D('',#59228,#22832,#22833);
#20431=AXIS2_PLACEMENT_3D('',#59229,#22834,#22835);
#20432=AXIS2_PLACEMENT_3D('',#59230,#22836,#22837);
#20433=AXIS2_PLACEMENT_3D('',#59232,#22838,#22839);
#20434=AXIS2_PLACEMENT_3D('',#59233,#22840,#22841);
#20435=AXIS2_PLACEMENT_3D('',#59234,#22842,#22843);
#20436=AXIS2_PLACEMENT_3D('',#59238,#22845,#22846);
#20437=AXIS2_PLACEMENT_3D('',#59240,#22848,#22849);
#20438=AXIS2_PLACEMENT_3D('',#59241,#22850,#22851);
#20439=AXIS2_PLACEMENT_3D('',#59242,#22852,#22853);
#20440=AXIS2_PLACEMENT_3D('',#59244,#22854,#22855);
#20441=AXIS2_PLACEMENT_3D('',#59246,#22856,#22857);
#20442=AXIS2_PLACEMENT_3D('',#59248,#22858,#22859);
#20443=AXIS2_PLACEMENT_3D('',#59249,#22860,#22861);
#20444=AXIS2_PLACEMENT_3D('',#59250,#22862,#22863);
#20445=AXIS2_PLACEMENT_3D('',#59297,#22886,#22887);
#20446=AXIS2_PLACEMENT_3D('',#59300,#22889,#22890);
#20447=AXIS2_PLACEMENT_3D('',#59305,#22892,#22893);
#20448=AXIS2_PLACEMENT_3D('',#59308,#22895,#22896);
#20449=AXIS2_PLACEMENT_3D('',#59312,#22898,#22899);
#20450=AXIS2_PLACEMENT_3D('',#59316,#22901,#22902);
#20451=AXIS2_PLACEMENT_3D('',#59320,#22904,#22905);
#20452=AXIS2_PLACEMENT_3D('',#59322,#22907,#22908);
#20453=AXIS2_PLACEMENT_3D('',#59324,#22909,#22910);
#20454=AXIS2_PLACEMENT_3D('',#59327,#22911,#22912);
#20455=AXIS2_PLACEMENT_3D('',#59330,#22914,#22915);
#20456=AXIS2_PLACEMENT_3D('',#59332,#22917,#22918);
#20457=AXIS2_PLACEMENT_3D('',#59335,#22920,#22921);
#20458=AXIS2_PLACEMENT_3D('',#59338,#22923,#22924);
#20459=AXIS2_PLACEMENT_3D('',#59339,#22925,#22926);
#20460=AXIS2_PLACEMENT_3D('',#59343,#22928,#22929);
#20461=AXIS2_PLACEMENT_3D('',#59344,#22930,#22931);
#20462=AXIS2_PLACEMENT_3D('',#59345,#22932,#22933);
#20463=AXIS2_PLACEMENT_3D('',#59347,#22934,#22935);
#20464=AXIS2_PLACEMENT_3D('',#59349,#22936,#22937);
#20465=AXIS2_PLACEMENT_3D('',#59350,#22938,#22939);
#20466=AXIS2_PLACEMENT_3D('',#59351,#22940,#22941);
#20467=AXIS2_PLACEMENT_3D('',#59355,#22943,#22944);
#20468=AXIS2_PLACEMENT_3D('',#59356,#22945,#22946);
#20469=AXIS2_PLACEMENT_3D('',#59357,#22947,#22948);
#20470=AXIS2_PLACEMENT_3D('',#59358,#22949,#22950);
#20471=AXIS2_PLACEMENT_3D('',#59359,#22951,#22952);
#20472=AXIS2_PLACEMENT_3D('',#59361,#22953,#22954);
#20473=AXIS2_PLACEMENT_3D('',#59364,#22956,#22957);
#20474=AXIS2_PLACEMENT_3D('',#59365,#22958,#22959);
#20475=AXIS2_PLACEMENT_3D('',#59367,#22960,#22961);
#20476=AXIS2_PLACEMENT_3D('',#59368,#22962,#22963);
#20477=AXIS2_PLACEMENT_3D('',#59369,#22964,#22965);
#20478=AXIS2_PLACEMENT_3D('',#59371,#22966,#22967);
#20479=AXIS2_PLACEMENT_3D('',#59373,#22969,#22970);
#20480=AXIS2_PLACEMENT_3D('',#59374,#22971,#22972);
#20481=AXIS2_PLACEMENT_3D('',#59375,#22973,#22974);
#20482=AXIS2_PLACEMENT_3D('',#59379,#22976,#22977);
#20483=AXIS2_PLACEMENT_3D('',#59381,#22979,#22980);
#20484=AXIS2_PLACEMENT_3D('',#59385,#22983,#22984);
#20485=AXIS2_PLACEMENT_3D('',#59388,#22986,#22987);
#20486=AXIS2_PLACEMENT_3D('',#59389,#22988,#22989);
#20487=AXIS2_PLACEMENT_3D('',#59390,#22990,#22991);
#20488=AXIS2_PLACEMENT_3D('',#59391,#22992,#22993);
#20489=AXIS2_PLACEMENT_3D('',#59393,#22994,#22995);
#20490=AXIS2_PLACEMENT_3D('',#59394,#22996,#22997);
#20491=AXIS2_PLACEMENT_3D('',#59395,#22998,#22999);
#20492=AXIS2_PLACEMENT_3D('',#59396,#23000,#23001);
#20493=AXIS2_PLACEMENT_3D('',#59398,#23002,#23003);
#20494=AXIS2_PLACEMENT_3D('',#59399,#23004,#23005);
#20495=AXIS2_PLACEMENT_3D('',#59400,#23006,#23007);
#20496=AXIS2_PLACEMENT_3D('',#59402,#23009,#23010);
#20497=AXIS2_PLACEMENT_3D('',#59405,#23012,#23013);
#20498=AXIS2_PLACEMENT_3D('',#59406,#23014,#23015);
#20499=AXIS2_PLACEMENT_3D('',#59408,#23016,#23017);
#20500=AXIS2_PLACEMENT_3D('',#59409,#23018,#23019);
#20501=AXIS2_PLACEMENT_3D('',#59410,#23020,#23021);
#20502=AXIS2_PLACEMENT_3D('',#59412,#23022,#23023);
#20503=AXIS2_PLACEMENT_3D('',#59414,#23024,#23025);
#20504=AXIS2_PLACEMENT_3D('',#59416,#23027,#23028);
#20505=AXIS2_PLACEMENT_3D('',#59418,#23029,#23030);
#20506=AXIS2_PLACEMENT_3D('',#59419,#23031,#23032);
#20507=AXIS2_PLACEMENT_3D('',#59420,#23033,#23034);
#20508=AXIS2_PLACEMENT_3D('',#59422,#23035,#23036);
#20509=AXIS2_PLACEMENT_3D('',#59424,#23038,#23039);
#20510=AXIS2_PLACEMENT_3D('',#59427,#23040,#23041);
#20511=AXIS2_PLACEMENT_3D('',#59428,#23042,#23043);
#20512=AXIS2_PLACEMENT_3D('',#59429,#23044,#23045);
#20513=AXIS2_PLACEMENT_3D('',#59430,#23046,#23047);
#20514=AXIS2_PLACEMENT_3D('',#59432,#23048,#23049);
#20515=AXIS2_PLACEMENT_3D('',#59434,#23050,#23051);
#20516=AXIS2_PLACEMENT_3D('',#59435,#23052,#23053);
#20517=AXIS2_PLACEMENT_3D('',#59436,#23054,#23055);
#20518=AXIS2_PLACEMENT_3D('',#59438,#23057,#23058);
#20519=AXIS2_PLACEMENT_3D('',#59441,#23059,#23060);
#20520=AXIS2_PLACEMENT_3D('',#59442,#23061,#23062);
#20521=AXIS2_PLACEMENT_3D('',#59443,#23063,#23064);
#20522=AXIS2_PLACEMENT_3D('',#59444,#23065,#23066);
#20523=AXIS2_PLACEMENT_3D('',#59446,#23068,#23069);
#20524=AXIS2_PLACEMENT_3D('',#59449,#23070,#23071);
#20525=AXIS2_PLACEMENT_3D('',#59450,#23072,#23073);
#20526=AXIS2_PLACEMENT_3D('',#59451,#23074,#23075);
#20527=AXIS2_PLACEMENT_3D('',#59452,#23076,#23077);
#20528=AXIS2_PLACEMENT_3D('',#59454,#23079,#23080);
#20529=AXIS2_PLACEMENT_3D('',#59456,#23081,#23082);
#20530=AXIS2_PLACEMENT_3D('',#59458,#23084,#23085);
#20531=AXIS2_PLACEMENT_3D('',#59460,#23086,#23087);
#20532=AXIS2_PLACEMENT_3D('',#59461,#23088,#23089);
#20533=AXIS2_PLACEMENT_3D('',#59462,#23090,#23091);
#20534=AXIS2_PLACEMENT_3D('',#59465,#23092,#23093);
#20535=AXIS2_PLACEMENT_3D('',#59468,#23096,#23097);
#20536=AXIS2_PLACEMENT_3D('',#59470,#23098,#23099);
#20537=AXIS2_PLACEMENT_3D('',#59471,#23100,#23101);
#20538=AXIS2_PLACEMENT_3D('',#59472,#23102,#23103);
#20539=AXIS2_PLACEMENT_3D('',#59475,#23104,#23105);
#20540=AXIS2_PLACEMENT_3D('',#59478,#23108,#23109);
#20541=AXIS2_PLACEMENT_3D('',#59480,#23110,#23111);
#20542=AXIS2_PLACEMENT_3D('',#59481,#23112,#23113);
#20543=AXIS2_PLACEMENT_3D('',#59482,#23114,#23115);
#20544=AXIS2_PLACEMENT_3D('',#59485,#23116,#23117);
#20545=AXIS2_PLACEMENT_3D('',#59488,#23120,#23121);
#20546=AXIS2_PLACEMENT_3D('',#59490,#23122,#23123);
#20547=AXIS2_PLACEMENT_3D('',#59491,#23124,#23125);
#20548=AXIS2_PLACEMENT_3D('',#59492,#23126,#23127);
#20549=AXIS2_PLACEMENT_3D('',#59494,#23129,#23130);
#20550=AXIS2_PLACEMENT_3D('',#59496,#23132,#23133);
#20551=AXIS2_PLACEMENT_3D('',#59498,#23135,#23136);
#20552=AXIS2_PLACEMENT_3D('',#59502,#23138,#23139);
#20553=AXIS2_PLACEMENT_3D('',#59504,#23141,#23142);
#20554=AXIS2_PLACEMENT_3D('',#59506,#23144,#23145);
#20555=AXIS2_PLACEMENT_3D('',#59508,#23146,#23147);
#20556=AXIS2_PLACEMENT_3D('',#59510,#23148,#23149);
#20557=AXIS2_PLACEMENT_3D('',#59511,#23150,#23151);
#20558=AXIS2_PLACEMENT_3D('',#59512,#23152,#23153);
#20559=AXIS2_PLACEMENT_3D('',#59515,#23154,#23155);
#20560=AXIS2_PLACEMENT_3D('',#59517,#23156,#23157);
#20561=AXIS2_PLACEMENT_3D('',#59518,#23158,#23159);
#20562=AXIS2_PLACEMENT_3D('',#59519,#23160,#23161);
#20563=AXIS2_PLACEMENT_3D('',#59522,#23164,#23165);
#20564=AXIS2_PLACEMENT_3D('',#59524,#23166,#23167);
#20565=AXIS2_PLACEMENT_3D('',#59525,#23168,#23169);
#20566=AXIS2_PLACEMENT_3D('',#59526,#23170,#23171);
#20567=AXIS2_PLACEMENT_3D('',#59528,#23172,#23173);
#20568=AXIS2_PLACEMENT_3D('',#59529,#23174,#23175);
#20569=AXIS2_PLACEMENT_3D('',#59530,#23176,#23177);
#20570=AXIS2_PLACEMENT_3D('',#59532,#23178,#23179);
#20571=AXIS2_PLACEMENT_3D('',#59534,#23181,#23182);
#20572=AXIS2_PLACEMENT_3D('',#59536,#23183,#23184);
#20573=AXIS2_PLACEMENT_3D('',#59537,#23185,#23186);
#20574=AXIS2_PLACEMENT_3D('',#59538,#23187,#23188);
#20575=AXIS2_PLACEMENT_3D('',#59539,#23189,#23190);
#20576=AXIS2_PLACEMENT_3D('',#59540,#23191,#23192);
#20577=AXIS2_PLACEMENT_3D('',#59541,#23193,#23194);
#20578=AXIS2_PLACEMENT_3D('',#59542,#23195,#23196);
#20579=AXIS2_PLACEMENT_3D('',#59544,#23197,#23198);
#20580=AXIS2_PLACEMENT_3D('',#59545,#23199,#23200);
#20581=AXIS2_PLACEMENT_3D('',#59546,#23201,#23202);
#20582=AXIS2_PLACEMENT_3D('',#59547,#23203,#23204);
#20583=AXIS2_PLACEMENT_3D('',#59548,#23205,#23206);
#20584=AXIS2_PLACEMENT_3D('',#59549,#23207,#23208);
#20585=AXIS2_PLACEMENT_3D('',#59551,#23209,#23210);
#20586=AXIS2_PLACEMENT_3D('',#59553,#23211,#23212);
#20587=AXIS2_PLACEMENT_3D('',#59554,#23213,#23214);
#20588=AXIS2_PLACEMENT_3D('',#59555,#23215,#23216);
#20589=AXIS2_PLACEMENT_3D('',#59558,#23218,#23219);
#20590=AXIS2_PLACEMENT_3D('',#59560,#23221,#23222);
#20591=AXIS2_PLACEMENT_3D('',#59562,#23224,#23225);
#20592=AXIS2_PLACEMENT_3D('',#59564,#23227,#23228);
#20593=AXIS2_PLACEMENT_3D('',#59565,#23229,#23230);
#20594=AXIS2_PLACEMENT_3D('',#59566,#23231,#23232);
#20595=AXIS2_PLACEMENT_3D('',#59569,#23234,#23235);
#20596=AXIS2_PLACEMENT_3D('',#59570,#23236,#23237);
#20597=AXIS2_PLACEMENT_3D('',#59572,#23238,#23239);
#20598=AXIS2_PLACEMENT_3D('',#59574,#23240,#23241);
#20599=AXIS2_PLACEMENT_3D('',#59575,#23242,#23243);
#20600=AXIS2_PLACEMENT_3D('',#59576,#23244,#23245);
#20601=AXIS2_PLACEMENT_3D('',#59580,#23247,#23248);
#20602=AXIS2_PLACEMENT_3D('',#59581,#23249,#23250);
#20603=AXIS2_PLACEMENT_3D('',#59582,#23251,#23252);
#20604=AXIS2_PLACEMENT_3D('',#59585,#23253,#23254);
#20605=AXIS2_PLACEMENT_3D('',#59586,#23255,#23256);
#20606=AXIS2_PLACEMENT_3D('',#59587,#23257,#23258);
#20607=AXIS2_PLACEMENT_3D('',#59588,#23259,#23260);
#20608=AXIS2_PLACEMENT_3D('',#59590,#23262,#23263);
#20609=AXIS2_PLACEMENT_3D('',#59593,#23264,#23265);
#20610=AXIS2_PLACEMENT_3D('',#59594,#23266,#23267);
#20611=AXIS2_PLACEMENT_3D('',#59595,#23268,#23269);
#20612=AXIS2_PLACEMENT_3D('',#59596,#23270,#23271);
#20613=AXIS2_PLACEMENT_3D('',#59598,#23273,#23274);
#20614=AXIS2_PLACEMENT_3D('',#59601,#23275,#23276);
#20615=AXIS2_PLACEMENT_3D('',#59602,#23277,#23278);
#20616=AXIS2_PLACEMENT_3D('',#59603,#23279,#23280);
#20617=AXIS2_PLACEMENT_3D('',#59604,#23281,#23282);
#20618=AXIS2_PLACEMENT_3D('',#59606,#23284,#23285);
#20619=AXIS2_PLACEMENT_3D('',#59609,#23286,#23287);
#20620=AXIS2_PLACEMENT_3D('',#59610,#23288,#23289);
#20621=AXIS2_PLACEMENT_3D('',#59611,#23290,#23291);
#20622=AXIS2_PLACEMENT_3D('',#59612,#23292,#23293);
#20623=AXIS2_PLACEMENT_3D('',#59614,#23295,#23296);
#20624=AXIS2_PLACEMENT_3D('',#59617,#23298,#23299);
#20625=AXIS2_PLACEMENT_3D('',#59618,#23300,#23301);
#20626=AXIS2_PLACEMENT_3D('',#59620,#23302,#23303);
#20627=AXIS2_PLACEMENT_3D('',#59622,#23305,#23306);
#20628=AXIS2_PLACEMENT_3D('',#59625,#23307,#23308);
#20629=AXIS2_PLACEMENT_3D('',#59626,#23309,#23310);
#20630=AXIS2_PLACEMENT_3D('',#59627,#23311,#23312);
#20631=AXIS2_PLACEMENT_3D('',#59628,#23313,#23314);
#20632=AXIS2_PLACEMENT_3D('',#59630,#23316,#23317);
#20633=AXIS2_PLACEMENT_3D('',#59632,#23319,#23320);
#20634=AXIS2_PLACEMENT_3D('',#59635,#23321,#23322);
#20635=AXIS2_PLACEMENT_3D('',#59638,#23325,#23326);
#20636=AXIS2_PLACEMENT_3D('',#59640,#23327,#23328);
#20637=AXIS2_PLACEMENT_3D('',#59641,#23329,#23330);
#20638=AXIS2_PLACEMENT_3D('',#59642,#23331,#23332);
#20639=AXIS2_PLACEMENT_3D('',#59645,#23333,#23334);
#20640=AXIS2_PLACEMENT_3D('',#59648,#23337,#23338);
#20641=AXIS2_PLACEMENT_3D('',#59650,#23339,#23340);
#20642=AXIS2_PLACEMENT_3D('',#59651,#23341,#23342);
#20643=AXIS2_PLACEMENT_3D('',#59652,#23343,#23344);
#20644=AXIS2_PLACEMENT_3D('',#59655,#23345,#23346);
#20645=AXIS2_PLACEMENT_3D('',#59658,#23349,#23350);
#20646=AXIS2_PLACEMENT_3D('',#59660,#23351,#23352);
#20647=AXIS2_PLACEMENT_3D('',#59661,#23353,#23354);
#20648=AXIS2_PLACEMENT_3D('',#59662,#23355,#23356);
#20649=AXIS2_PLACEMENT_3D('',#59665,#23357,#23358);
#20650=AXIS2_PLACEMENT_3D('',#59668,#23361,#23362);
#20651=AXIS2_PLACEMENT_3D('',#59670,#23363,#23364);
#20652=AXIS2_PLACEMENT_3D('',#59671,#23365,#23366);
#20653=AXIS2_PLACEMENT_3D('',#59672,#23367,#23368);
#20654=AXIS2_PLACEMENT_3D('',#59675,#23369,#23370);
#20655=AXIS2_PLACEMENT_3D('',#59678,#23373,#23374);
#20656=AXIS2_PLACEMENT_3D('',#59680,#23375,#23376);
#20657=AXIS2_PLACEMENT_3D('',#59681,#23377,#23378);
#20658=AXIS2_PLACEMENT_3D('',#59682,#23379,#23380);
#20659=AXIS2_PLACEMENT_3D('',#59685,#23382,#23383);
#20660=AXIS2_PLACEMENT_3D('',#59686,#23384,#23385);
#20661=AXIS2_PLACEMENT_3D('',#59687,#23386,#23387);
#20662=AXIS2_PLACEMENT_3D('',#59688,#23388,#23389);
#20663=AXIS2_PLACEMENT_3D('',#59690,#23391,#23392);
#20664=AXIS2_PLACEMENT_3D('',#59693,#23395,#23396);
#20665=AXIS2_PLACEMENT_3D('',#59695,#23398,#23399);
#20666=AXIS2_PLACEMENT_3D('',#59697,#23401,#23402);
#20667=AXIS2_PLACEMENT_3D('',#59699,#23404,#23405);
#20668=AXIS2_PLACEMENT_3D('',#59703,#23407,#23408);
#20669=AXIS2_PLACEMENT_3D('',#59705,#23410,#23411);
#20670=AXIS2_PLACEMENT_3D('',#59707,#23413,#23414);
#20671=AXIS2_PLACEMENT_3D('',#59711,#23417,#23418);
#20672=AXIS2_PLACEMENT_3D('',#59713,#23420,#23421);
#20673=AXIS2_PLACEMENT_3D('',#59716,#23423,#23424);
#20674=AXIS2_PLACEMENT_3D('',#59717,#23425,#23426);
#20675=AXIS2_PLACEMENT_3D('',#59721,#23428,#23429);
#20676=AXIS2_PLACEMENT_3D('',#59723,#23431,#23432);
#20677=AXIS2_PLACEMENT_3D('',#59725,#23434,#23435);
#20678=AXIS2_PLACEMENT_3D('',#59727,#23436,#23437);
#20679=AXIS2_PLACEMENT_3D('',#59728,#23438,#23439);
#20680=AXIS2_PLACEMENT_3D('',#59729,#23440,#23441);
#20681=AXIS2_PLACEMENT_3D('',#59735,#23444,#23445);
#20682=AXIS2_PLACEMENT_3D('',#59759,#23459,#23460);
#20683=AXIS2_PLACEMENT_3D('',#59763,#23462,#23463);
#20684=AXIS2_PLACEMENT_3D('',#59766,#23465,#23466);
#20685=AXIS2_PLACEMENT_3D('',#59771,#23468,#23469);
#20686=AXIS2_PLACEMENT_3D('',#59774,#23471,#23472);
#20687=AXIS2_PLACEMENT_3D('',#59776,#23473,#23474);
#20688=AXIS2_PLACEMENT_3D('',#59779,#23476,#23477);
#20689=AXIS2_PLACEMENT_3D('',#59781,#23478,#23479);
#20690=AXIS2_PLACEMENT_3D('',#59782,#23480,#23481);
#20691=AXIS2_PLACEMENT_3D('',#59783,#23482,#23483);
#20692=AXIS2_PLACEMENT_3D('',#59784,#23484,#23485);
#20693=AXIS2_PLACEMENT_3D('',#59786,#23486,#23487);
#20694=AXIS2_PLACEMENT_3D('',#59788,#23489,#23490);
#20695=AXIS2_PLACEMENT_3D('',#59790,#23492,#23493);
#20696=AXIS2_PLACEMENT_3D('',#59792,#23495,#23496);
#20697=AXIS2_PLACEMENT_3D('',#59794,#23498,#23499);
#20698=AXIS2_PLACEMENT_3D('',#59795,#23500,#23501);
#20699=AXIS2_PLACEMENT_3D('',#59796,#23502,#23503);
#20700=AXIS2_PLACEMENT_3D('',#59797,#23504,#23505);
#20701=AXIS2_PLACEMENT_3D('',#59798,#23506,#23507);
#20702=AXIS2_PLACEMENT_3D('',#59799,#23508,#23509);
#20703=AXIS2_PLACEMENT_3D('',#59801,#23511,#23512);
#20704=AXIS2_PLACEMENT_3D('',#59802,#23513,#23514);
#20705=AXIS2_PLACEMENT_3D('',#59804,#23515,#23516);
#20706=AXIS2_PLACEMENT_3D('',#59806,#23517,#23518);
#20707=AXIS2_PLACEMENT_3D('',#59807,#23519,#23520);
#20708=AXIS2_PLACEMENT_3D('',#59808,#23521,#23522);
#20709=AXIS2_PLACEMENT_3D('',#59810,#23524,#23525);
#20710=AXIS2_PLACEMENT_3D('',#59811,#23526,#23527);
#20711=AXIS2_PLACEMENT_3D('',#59812,#23528,#23529);
#20712=AXIS2_PLACEMENT_3D('',#59814,#23531,#23532);
#20713=AXIS2_PLACEMENT_3D('',#59816,#23534,#23535);
#20714=AXIS2_PLACEMENT_3D('',#59818,#23536,#23537);
#20715=AXIS2_PLACEMENT_3D('',#59819,#23538,#23539);
#20716=AXIS2_PLACEMENT_3D('',#59820,#23540,#23541);
#20717=AXIS2_PLACEMENT_3D('',#59823,#23542,#23543);
#20718=AXIS2_PLACEMENT_3D('',#59824,#23544,#23545);
#20719=AXIS2_PLACEMENT_3D('',#59825,#23546,#23547);
#20720=AXIS2_PLACEMENT_3D('',#59826,#23548,#23549);
#20721=AXIS2_PLACEMENT_3D('',#59828,#23551,#23552);
#20722=AXIS2_PLACEMENT_3D('',#59830,#23553,#23554);
#20723=AXIS2_PLACEMENT_3D('',#59832,#23555,#23556);
#20724=AXIS2_PLACEMENT_3D('',#59833,#23557,#23558);
#20725=AXIS2_PLACEMENT_3D('',#59834,#23559,#23560);
#20726=AXIS2_PLACEMENT_3D('',#59835,#23561,#23562);
#20727=AXIS2_PLACEMENT_3D('',#59836,#23563,#23564);
#20728=AXIS2_PLACEMENT_3D('',#59839,#23565,#23566);
#20729=AXIS2_PLACEMENT_3D('',#59842,#23569,#23570);
#20730=AXIS2_PLACEMENT_3D('',#59843,#23571,#23572);
#20731=AXIS2_PLACEMENT_3D('',#59844,#23573,#23574);
#20732=AXIS2_PLACEMENT_3D('',#59845,#23575,#23576);
#20733=AXIS2_PLACEMENT_3D('',#59848,#23577,#23578);
#20734=AXIS2_PLACEMENT_3D('',#59849,#23579,#23580);
#20735=AXIS2_PLACEMENT_3D('',#59850,#23581,#23582);
#20736=AXIS2_PLACEMENT_3D('',#59851,#23583,#23584);
#20737=AXIS2_PLACEMENT_3D('',#59854,#23587,#23588);
#20738=AXIS2_PLACEMENT_3D('',#59855,#23589,#23590);
#20739=AXIS2_PLACEMENT_3D('',#59856,#23591,#23592);
#20740=AXIS2_PLACEMENT_3D('',#59857,#23593,#23594);
#20741=AXIS2_PLACEMENT_3D('',#59858,#23595,#23596);
#20742=AXIS2_PLACEMENT_3D('',#59859,#23597,#23598);
#20743=AXIS2_PLACEMENT_3D('',#59861,#23599,#23600);
#20744=AXIS2_PLACEMENT_3D('',#59862,#23601,#23602);
#20745=AXIS2_PLACEMENT_3D('',#59863,#23603,#23604);
#20746=AXIS2_PLACEMENT_3D('',#59865,#23606,#23607);
#20747=AXIS2_PLACEMENT_3D('',#59867,#23608,#23609);
#20748=AXIS2_PLACEMENT_3D('',#59868,#23610,#23611);
#20749=AXIS2_PLACEMENT_3D('',#59869,#23612,#23613);
#20750=AXIS2_PLACEMENT_3D('',#59871,#23614,#23615);
#20751=AXIS2_PLACEMENT_3D('',#59872,#23616,#23617);
#20752=AXIS2_PLACEMENT_3D('',#59873,#23618,#23619);
#20753=AXIS2_PLACEMENT_3D('',#59875,#23620,#23621);
#20754=AXIS2_PLACEMENT_3D('',#59876,#23622,#23623);
#20755=AXIS2_PLACEMENT_3D('',#59877,#23624,#23625);
#20756=AXIS2_PLACEMENT_3D('',#59880,#23626,#23627);
#20757=AXIS2_PLACEMENT_3D('',#59881,#23628,#23629);
#20758=AXIS2_PLACEMENT_3D('',#59882,#23630,#23631);
#20759=AXIS2_PLACEMENT_3D('',#59883,#23632,#23633);
#20760=AXIS2_PLACEMENT_3D('',#59886,#23636,#23637);
#20761=AXIS2_PLACEMENT_3D('',#59888,#23639,#23640);
#20762=AXIS2_PLACEMENT_3D('',#59891,#23642,#23643);
#20763=AXIS2_PLACEMENT_3D('',#59893,#23645,#23646);
#20764=AXIS2_PLACEMENT_3D('',#59894,#23647,#23648);
#20765=AXIS2_PLACEMENT_3D('',#59895,#23649,#23650);
#20766=AXIS2_PLACEMENT_3D('',#59897,#23652,#23653);
#20767=AXIS2_PLACEMENT_3D('',#59898,#23654,#23655);
#20768=AXIS2_PLACEMENT_3D('',#59900,#23656,#23657);
#20769=AXIS2_PLACEMENT_3D('',#59902,#23659,#23660);
#20770=AXIS2_PLACEMENT_3D('',#59905,#23661,#23662);
#20771=AXIS2_PLACEMENT_3D('',#59906,#23663,#23664);
#20772=AXIS2_PLACEMENT_3D('',#59907,#23665,#23666);
#20773=AXIS2_PLACEMENT_3D('',#59908,#23667,#23668);
#20774=AXIS2_PLACEMENT_3D('',#59910,#23669,#23670);
#20775=AXIS2_PLACEMENT_3D('',#59911,#23671,#23672);
#20776=AXIS2_PLACEMENT_3D('',#59912,#23673,#23674);
#20777=AXIS2_PLACEMENT_3D('',#59914,#23676,#23677);
#20778=AXIS2_PLACEMENT_3D('',#59917,#23679,#23680);
#20779=AXIS2_PLACEMENT_3D('',#59918,#23681,#23682);
#20780=AXIS2_PLACEMENT_3D('',#59921,#23683,#23684);
#20781=AXIS2_PLACEMENT_3D('',#59922,#23685,#23686);
#20782=AXIS2_PLACEMENT_3D('',#59923,#23687,#23688);
#20783=AXIS2_PLACEMENT_3D('',#59924,#23689,#23690);
#20784=AXIS2_PLACEMENT_3D('',#59926,#23692,#23693);
#20785=AXIS2_PLACEMENT_3D('',#59929,#23695,#23696);
#20786=AXIS2_PLACEMENT_3D('',#59930,#23697,#23698);
#20787=AXIS2_PLACEMENT_3D('',#59932,#23699,#23700);
#20788=AXIS2_PLACEMENT_3D('',#59934,#23702,#23703);
#20789=AXIS2_PLACEMENT_3D('',#59937,#23704,#23705);
#20790=AXIS2_PLACEMENT_3D('',#59938,#23706,#23707);
#20791=AXIS2_PLACEMENT_3D('',#59939,#23708,#23709);
#20792=AXIS2_PLACEMENT_3D('',#59940,#23710,#23711);
#20793=AXIS2_PLACEMENT_3D('',#59942,#23713,#23714);
#20794=AXIS2_PLACEMENT_3D('',#59945,#23715,#23716);
#20795=AXIS2_PLACEMENT_3D('',#59946,#23717,#23718);
#20796=AXIS2_PLACEMENT_3D('',#59947,#23719,#23720);
#20797=AXIS2_PLACEMENT_3D('',#59948,#23721,#23722);
#20798=AXIS2_PLACEMENT_3D('',#59950,#23724,#23725);
#20799=AXIS2_PLACEMENT_3D('',#59953,#23726,#23727);
#20800=AXIS2_PLACEMENT_3D('',#59954,#23728,#23729);
#20801=AXIS2_PLACEMENT_3D('',#59955,#23730,#23731);
#20802=AXIS2_PLACEMENT_3D('',#59956,#23732,#23733);
#20803=AXIS2_PLACEMENT_3D('',#59958,#23735,#23736);
#20804=AXIS2_PLACEMENT_3D('',#59960,#23738,#23739);
#20805=AXIS2_PLACEMENT_3D('',#59963,#23740,#23741);
#20806=AXIS2_PLACEMENT_3D('',#59966,#23744,#23745);
#20807=AXIS2_PLACEMENT_3D('',#59967,#23746,#23747);
#20808=AXIS2_PLACEMENT_3D('',#59969,#23749,#23750);
#20809=AXIS2_PLACEMENT_3D('',#59972,#23751,#23752);
#20810=AXIS2_PLACEMENT_3D('',#59975,#23755,#23756);
#20811=AXIS2_PLACEMENT_3D('',#59976,#23757,#23758);
#20812=AXIS2_PLACEMENT_3D('',#59977,#23759,#23760);
#20813=AXIS2_PLACEMENT_3D('',#59978,#23761,#23762);
#20814=AXIS2_PLACEMENT_3D('',#59981,#23763,#23764);
#20815=AXIS2_PLACEMENT_3D('',#59984,#23767,#23768);
#20816=AXIS2_PLACEMENT_3D('',#59985,#23769,#23770);
#20817=AXIS2_PLACEMENT_3D('',#59986,#23771,#23772);
#20818=AXIS2_PLACEMENT_3D('',#59987,#23773,#23774);
#20819=AXIS2_PLACEMENT_3D('',#59990,#23775,#23776);
#20820=AXIS2_PLACEMENT_3D('',#59993,#23779,#23780);
#20821=AXIS2_PLACEMENT_3D('',#59994,#23781,#23782);
#20822=AXIS2_PLACEMENT_3D('',#59995,#23783,#23784);
#20823=AXIS2_PLACEMENT_3D('',#59996,#23785,#23786);
#20824=AXIS2_PLACEMENT_3D('',#59999,#23787,#23788);
#20825=AXIS2_PLACEMENT_3D('',#60002,#23791,#23792);
#20826=AXIS2_PLACEMENT_3D('',#60003,#23793,#23794);
#20827=AXIS2_PLACEMENT_3D('',#60004,#23795,#23796);
#20828=AXIS2_PLACEMENT_3D('',#60005,#23797,#23798);
#20829=AXIS2_PLACEMENT_3D('',#60008,#23800,#23801);
#20830=AXIS2_PLACEMENT_3D('',#60010,#23803,#23804);
#20831=AXIS2_PLACEMENT_3D('',#60011,#23805,#23806);
#20832=AXIS2_PLACEMENT_3D('',#60012,#23807,#23808);
#20833=AXIS2_PLACEMENT_3D('',#60013,#23809,#23810);
#20834=AXIS2_PLACEMENT_3D('',#60014,#23811,#23812);
#20835=AXIS2_PLACEMENT_3D('',#60016,#23813,#23814);
#20836=AXIS2_PLACEMENT_3D('',#60018,#23816,#23817);
#20837=AXIS2_PLACEMENT_3D('',#60021,#23819,#23820);
#20838=AXIS2_PLACEMENT_3D('',#60022,#23821,#23822);
#20839=AXIS2_PLACEMENT_3D('',#60024,#23824,#23825);
#20840=AXIS2_PLACEMENT_3D('',#60026,#23827,#23828);
#20841=AXIS2_PLACEMENT_3D('',#60027,#23829,#23830);
#20842=AXIS2_PLACEMENT_3D('',#60030,#23832,#23833);
#20843=AXIS2_PLACEMENT_3D('',#60031,#23834,#23835);
#20844=AXIS2_PLACEMENT_3D('',#60033,#23837,#23838);
#20845=AXIS2_PLACEMENT_3D('',#60037,#23841,#23842);
#20846=AXIS2_PLACEMENT_3D('',#60039,#23844,#23845);
#20847=AXIS2_PLACEMENT_3D('',#60040,#23846,#23847);
#20848=AXIS2_PLACEMENT_3D('',#60041,#23848,#23849);
#20849=AXIS2_PLACEMENT_3D('',#60043,#23851,#23852);
#20850=AXIS2_PLACEMENT_3D('',#60044,#23853,#23854);
#20851=AXIS2_PLACEMENT_3D('',#60046,#23856,#23857);
#20852=AXIS2_PLACEMENT_3D('',#60047,#23858,#23859);
#20853=AXIS2_PLACEMENT_3D('',#60048,#23860,#23861);
#20854=AXIS2_PLACEMENT_3D('',#60049,#23862,#23863);
#20855=AXIS2_PLACEMENT_3D('',#60052,#23865,#23866);
#20856=AXIS2_PLACEMENT_3D('',#60053,#23867,#23868);
#20857=AXIS2_PLACEMENT_3D('',#60054,#23869,#23870);
#20858=AXIS2_PLACEMENT_3D('',#60055,#23871,#23872);
#20859=AXIS2_PLACEMENT_3D('',#60057,#23874,#23875);
#20860=AXIS2_PLACEMENT_3D('',#60059,#23877,#23878);
#20861=AXIS2_PLACEMENT_3D('',#60060,#23879,#23880);
#20862=AXIS2_PLACEMENT_3D('',#60061,#23881,#23882);
#20863=AXIS2_PLACEMENT_3D('',#60062,#23883,#23884);
#20864=AXIS2_PLACEMENT_3D('',#60063,#23885,#23886);
#20865=AXIS2_PLACEMENT_3D('',#60065,#23888,#23889);
#20866=AXIS2_PLACEMENT_3D('',#60066,#23890,#23891);
#20867=AXIS2_PLACEMENT_3D('',#60067,#23892,#23893);
#20868=AXIS2_PLACEMENT_3D('',#60068,#23894,#23895);
#20869=AXIS2_PLACEMENT_3D('',#60069,#23896,#23897);
#20870=AXIS2_PLACEMENT_3D('',#60070,#23898,#23899);
#20871=AXIS2_PLACEMENT_3D('',#60071,#23900,#23901);
#20872=AXIS2_PLACEMENT_3D('',#60072,#23902,#23903);
#20873=AXIS2_PLACEMENT_3D('',#60074,#23904,#23905);
#20874=AXIS2_PLACEMENT_3D('',#60075,#23906,#23907);
#20875=AXIS2_PLACEMENT_3D('',#60076,#23908,#23909);
#20876=AXIS2_PLACEMENT_3D('',#60077,#23910,#23911);
#20877=AXIS2_PLACEMENT_3D('',#60079,#23913,#23914);
#20878=AXIS2_PLACEMENT_3D('',#60080,#23915,#23916);
#20879=AXIS2_PLACEMENT_3D('',#60082,#23918,#23919);
#20880=AXIS2_PLACEMENT_3D('',#60083,#23920,#23921);
#20881=AXIS2_PLACEMENT_3D('',#60084,#23922,#23923);
#20882=AXIS2_PLACEMENT_3D('',#60087,#23924,#23925);
#20883=AXIS2_PLACEMENT_3D('',#60088,#23926,#23927);
#20884=AXIS2_PLACEMENT_3D('',#60089,#23928,#23929);
#20885=AXIS2_PLACEMENT_3D('',#60090,#23930,#23931);
#20886=AXIS2_PLACEMENT_3D('',#60093,#23932,#23933);
#20887=AXIS2_PLACEMENT_3D('',#60094,#23934,#23935);
#20888=AXIS2_PLACEMENT_3D('',#60096,#23937,#23938);
#20889=AXIS2_PLACEMENT_3D('',#60097,#23939,#23940);
#20890=AXIS2_PLACEMENT_3D('',#60098,#23941,#23942);
#20891=AXIS2_PLACEMENT_3D('',#60099,#23943,#23944);
#22633=DIRECTION('axis',(0.,0.,1.));
#22634=DIRECTION('refdir',(1.,0.,0.));
#22635=DIRECTION('center_axis',(0.,-1.,0.));
#22636=DIRECTION('ref_axis',(0.,0.,-1.));
#22637=DIRECTION('center_axis',(0.,1.,1.15415719212674E-15));
#22638=DIRECTION('ref_axis',(1.,0.,0.));
#22639=DIRECTION('center_axis',(-1.,0.,0.));
#22640=DIRECTION('ref_axis',(0.,0.,1.));
#22641=DIRECTION('center_axis',(0.,-1.,0.));
#22642=DIRECTION('ref_axis',(1.,0.,0.));
#22643=DIRECTION('center_axis',(0.,-1.,0.));
#22644=DIRECTION('ref_axis',(1.,0.,0.));
#22645=DIRECTION('center_axis',(0.,1.,1.15415719212674E-15));
#22646=DIRECTION('ref_axis',(1.,0.,0.));
#22647=DIRECTION('center_axis',(0.,1.,0.));
#22648=DIRECTION('ref_axis',(1.,0.,0.));
#22649=DIRECTION('center_axis',(0.,1.,0.));
#22650=DIRECTION('ref_axis',(1.,0.,0.));
#22651=DIRECTION('center_axis',(0.,1.,0.));
#22652=DIRECTION('ref_axis',(1.,0.,0.));
#22653=DIRECTION('',(0.,1.,0.));
#22654=DIRECTION('center_axis',(0.,1.,0.));
#22655=DIRECTION('ref_axis',(1.,0.,0.));
#22656=DIRECTION('',(-0.707106781186547,0.707106781186548,8.65956056235493E-17));
#22657=DIRECTION('center_axis',(0.,-1.,0.));
#22658=DIRECTION('ref_axis',(1.,0.,0.));
#22659=DIRECTION('center_axis',(0.,-1.,0.));
#22660=DIRECTION('ref_axis',(1.,0.,0.));
#22661=DIRECTION('center_axis',(0.,1.,0.));
#22662=DIRECTION('ref_axis',(-0.796497710072376,0.,0.60464154492514));
#22663=DIRECTION('center_axis',(0.,1.,0.));
#22664=DIRECTION('ref_axis',(-1.,0.,0.));
#22665=DIRECTION('',(0.,1.,0.));
#22666=DIRECTION('center_axis',(0.,-1.,0.));
#22667=DIRECTION('ref_axis',(-0.268817204301075,0.,0.963191211894998));
#22668=DIRECTION('',(0.,-1.,0.));
#22669=DIRECTION('center_axis',(0.,0.,1.));
#22670=DIRECTION('ref_axis',(1.,0.,0.));
#22671=DIRECTION('center_axis',(-0.963191211894997,0.,-0.268817204301076));
#22672=DIRECTION('ref_axis',(0.268817204301076,0.,-0.963191211894997));
#22673=DIRECTION('center_axis',(0.,0.,1.));
#22674=DIRECTION('ref_axis',(-0.707106781186544,0.707106781186551,0.));
#22675=DIRECTION('center_axis',(0.,0.,1.));
#22676=DIRECTION('ref_axis',(1.,0.,0.));
#22677=DIRECTION('center_axis',(0.,0.,1.));
#22678=DIRECTION('ref_axis',(-0.707106781186544,-0.707106781186551,0.));
#22679=DIRECTION('center_axis',(-0.963191211894997,0.,-0.268817204301076));
#22680=DIRECTION('ref_axis',(0.268817204301076,0.,-0.963191211894997));
#22681=DIRECTION('center_axis',(0.,0.,1.));
#22682=DIRECTION('ref_axis',(-0.707106781186545,0.70710678118655,0.));
#22683=DIRECTION('',(0.,0.,-1.));
#22684=DIRECTION('center_axis',(0.,0.,-1.));
#22685=DIRECTION('ref_axis',(-0.707106781186544,0.707106781186551,0.));
#22686=DIRECTION('',(0.,0.,1.));
#22687=DIRECTION('center_axis',(0.,-1.,0.));
#22688=DIRECTION('ref_axis',(0.707106781186548,0.,0.707106781186547));
#22689=DIRECTION('center_axis',(0.,-1.,0.));
#22690=DIRECTION('ref_axis',(0.707106781186547,0.,0.707106781186547));
#22691=DIRECTION('center_axis',(-0.268817204301076,0.,-0.963191211894997));
#22692=DIRECTION('ref_axis',(0.963191211894997,0.,-0.268817204301076));
#22693=DIRECTION('center_axis',(0.,1.,0.));
#22694=DIRECTION('ref_axis',(0.707106781186547,0.,0.707106781186547));
#22695=DIRECTION('center_axis',(0.,1.,0.));
#22696=DIRECTION('ref_axis',(1.,0.,0.));
#22697=DIRECTION('center_axis',(0.,1.,0.));
#22698=DIRECTION('ref_axis',(0.826936230559385,0.,0.562295714538387));
#22699=DIRECTION('',(0.,-1.,0.));
#22700=DIRECTION('center_axis',(0.,-1.,0.));
#22701=DIRECTION('ref_axis',(-0.796497710072379,0.,-0.604641544925138));
#22702=DIRECTION('center_axis',(0.,-1.,0.));
#22703=DIRECTION('ref_axis',(-1.,0.,0.));
#22704=DIRECTION('',(0.,-1.,0.));
#22705=DIRECTION('center_axis',(0.,1.,0.));
#22706=DIRECTION('ref_axis',(-0.268817204301076,0.,-0.963191211894997));
#22707=DIRECTION('',(0.,1.,0.));
#22708=DIRECTION('center_axis',(0.,0.,1.));
#22709=DIRECTION('ref_axis',(1.,0.,0.));
#22710=DIRECTION('center_axis',(-0.963191211894997,0.,0.268817204301076));
#22711=DIRECTION('ref_axis',(0.268817204301076,0.,0.963191211894997));
#22712=DIRECTION('center_axis',(0.,0.,-1.));
#22713=DIRECTION('ref_axis',(-0.707106781186544,-0.707106781186551,0.));
#22714=DIRECTION('center_axis',(0.,0.,1.));
#22715=DIRECTION('ref_axis',(1.,0.,0.));
#22716=DIRECTION('center_axis',(-0.963191211894997,0.,0.268817204301076));
#22717=DIRECTION('ref_axis',(0.268817204301076,0.,0.963191211894997));
#22718=DIRECTION('center_axis',(0.,-1.,0.));
#22719=DIRECTION('ref_axis',(0.,0.,-1.));
#22720=DIRECTION('center_axis',(0.,1.,0.));
#22721=DIRECTION('ref_axis',(0.707106781186547,0.,-0.707106781186548));
#22722=DIRECTION('center_axis',(-0.268817204301076,0.,0.963191211894997));
#22723=DIRECTION('ref_axis',(-0.963191211894997,0.,-0.268817204301076));
#22724=DIRECTION('center_axis',(0.,-1.,0.));
#22725=DIRECTION('ref_axis',(0.707106781186547,0.,-0.707106781186548));
#22726=DIRECTION('center_axis',(1.,0.,0.));
#22727=DIRECTION('ref_axis',(0.,0.,-1.));
#22728=DIRECTION('',(0.,0.,-1.));
#22729=DIRECTION('center_axis',(0.,1.,0.));
#22730=DIRECTION('ref_axis',(0.60464154492514,0.,0.796497710072376));
#22731=DIRECTION('center_axis',(0.,1.,0.));
#22732=DIRECTION('ref_axis',(0.,0.,1.));
#22733=DIRECTION('',(0.,1.,0.));
#22734=DIRECTION('center_axis',(0.,-1.,0.));
#22735=DIRECTION('ref_axis',(0.963191211894997,0.,0.268817204301076));
#22736=DIRECTION('',(0.,-1.,0.));
#22737=DIRECTION('center_axis',(0.321470784124458,-0.846950546350565,0.423475273175289));
#22738=DIRECTION('ref_axis',(0.512101486820596,0.531671676917698,0.674594170712776));
#22739=DIRECTION('center_axis',(1.,0.,0.));
#22740=DIRECTION('ref_axis',(0.,0.707106781186551,0.707106781186544));
#22741=DIRECTION('center_axis',(-0.321470784124453,-0.846950546350573,-0.423475273175278));
#22742=DIRECTION('ref_axis',(0.512101486820604,-0.531671676917688,0.674594170712778));
#22743=DIRECTION('center_axis',(1.,0.,0.));
#22744=DIRECTION('ref_axis',(0.,-0.707106781186551,0.707106781186544));
#22745=DIRECTION('center_axis',(-0.268817204301076,0.,0.963191211894997));
#22746=DIRECTION('ref_axis',(-0.963191211894997,0.,-0.268817204301076));
#22747=DIRECTION('center_axis',(1.,0.,0.));
#22748=DIRECTION('ref_axis',(0.,0.707106781186553,0.707106781186542));
#22749=DIRECTION('',(-1.,0.,0.));
#22750=DIRECTION('center_axis',(-1.,0.,0.));
#22751=DIRECTION('ref_axis',(0.,0.707106781186551,0.707106781186544));
#22752=DIRECTION('',(1.,0.,0.));
#22753=DIRECTION('center_axis',(0.,1.,0.));
#22754=DIRECTION('ref_axis',(1.,0.,0.));
#22755=DIRECTION('center_axis',(0.,1.,0.));
#22756=DIRECTION('ref_axis',(0.707106781186547,0.,-0.707106781186548));
#22757=DIRECTION('center_axis',(0.,-1.,0.));
#22758=DIRECTION('ref_axis',(-0.604641544925143,0.,0.796497710072374));
#22759=DIRECTION('center_axis',(0.,-1.,0.));
#22760=DIRECTION('ref_axis',(0.,0.,1.));
#22761=DIRECTION('',(0.,-1.,0.));
#22762=DIRECTION('center_axis',(0.,1.,0.));
#22763=DIRECTION('ref_axis',(-0.963191211894998,0.,0.268817204301074));
#22764=DIRECTION('',(0.,1.,0.));
#22765=DIRECTION('center_axis',(0.321470784124453,-0.846950546350573,-0.423475273175278));
#22766=DIRECTION('ref_axis',(-0.512101486820604,-0.531671676917688,0.674594170712778));
#22767=DIRECTION('center_axis',(0.268817204301076,0.,0.963191211894997));
#22768=DIRECTION('ref_axis',(0.963191211894997,0.,-0.268817204301076));
#22769=DIRECTION('center_axis',(-1.,0.,0.));
#22770=DIRECTION('ref_axis',(0.,-0.707106781186551,0.707106781186544));
#22771=DIRECTION('center_axis',(-0.32147078412446,-0.84695054635057,0.423475273175279));
#22772=DIRECTION('ref_axis',(-0.512101486820602,0.531671676917693,0.674594170712776));
#22773=DIRECTION('center_axis',(0.268817204301076,0.,0.963191211894997));
#22774=DIRECTION('ref_axis',(0.963191211894997,0.,-0.268817204301076));
#22775=DIRECTION('center_axis',(0.,-1.,0.));
#22776=DIRECTION('ref_axis',(0.,0.,-1.));
#22777=DIRECTION('center_axis',(0.,1.,0.));
#22778=DIRECTION('ref_axis',(-0.562295714538387,0.,-0.826936230559385));
#22779=DIRECTION('center_axis',(-0.963191211894995,1.98964699753618E-15,
-0.268817204301083));
#22780=DIRECTION('ref_axis',(1.84149810182896E-30,1.,7.40148683083437E-15));
#22781=DIRECTION('center_axis',(0.,-1.,0.));
#22782=DIRECTION('ref_axis',(-0.562295714538387,0.,-0.826936230559385));
#22783=DIRECTION('center_axis',(0.,0.,-1.));
#22784=DIRECTION('ref_axis',(-1.,0.,0.));
#22785=DIRECTION('',(-1.,0.,0.));
#22786=DIRECTION('center_axis',(0.,-1.,0.));
#22787=DIRECTION('ref_axis',(0.604641544925143,0.,-0.796497710072374));
#22788=DIRECTION('center_axis',(0.,-1.,0.));
#22789=DIRECTION('ref_axis',(0.,0.,-1.));
#22790=DIRECTION('',(0.,-1.,0.));
#22791=DIRECTION('center_axis',(0.,1.,0.));
#22792=DIRECTION('ref_axis',(0.963191211894997,0.,-0.268817204301076));
#22793=DIRECTION('',(0.,1.,0.));
#22794=DIRECTION('center_axis',(-0.321470784124453,-0.846950546350573,0.423475273175278));
#22795=DIRECTION('ref_axis',(0.512101486820604,-0.531671676917688,-0.674594170712778));
#22796=DIRECTION('center_axis',(-0.268817204301076,0.,-0.963191211894997));
#22797=DIRECTION('ref_axis',(-0.963191211894997,0.,0.268817204301076));
#22798=DIRECTION('center_axis',(1.,0.,0.));
#22799=DIRECTION('ref_axis',(0.,-0.70710678118655,-0.707106781186545));
#22800=DIRECTION('center_axis',(0.321470784124459,-0.846950546350569,-0.423475273175281));
#22801=DIRECTION('ref_axis',(0.512101486820603,0.531671676917694,-0.674594170712774));
#22802=DIRECTION('center_axis',(1.,0.,0.));
#22803=DIRECTION('ref_axis',(0.,0.70710678118655,-0.707106781186545));
#22804=DIRECTION('center_axis',(-0.268817204301076,0.,-0.963191211894997));
#22805=DIRECTION('ref_axis',(-0.963191211894997,0.,0.268817204301076));
#22806=DIRECTION('center_axis',(0.,-1.,0.));
#22807=DIRECTION('ref_axis',(0.707106781186548,0.,0.707106781186547));
#22808=DIRECTION('center_axis',(0.,1.,0.));
#22809=DIRECTION('ref_axis',(0.707106781186547,0.,0.707106781186547));
#22810=DIRECTION('center_axis',(-0.963191211894997,0.,-0.268817204301078));
#22811=DIRECTION('ref_axis',(0.268817204301078,0.,-0.963191211894997));
#22812=DIRECTION('center_axis',(0.,-1.,0.));
#22813=DIRECTION('ref_axis',(0.707106781186547,0.,0.707106781186547));
#22814=DIRECTION('center_axis',(-1.,0.,0.));
#22815=DIRECTION('ref_axis',(0.,0.70710678118655,-0.707106781186545));
#22816=DIRECTION('',(-1.,0.,0.));
#22817=DIRECTION('center_axis',(-1.,0.,0.));
#22818=DIRECTION('ref_axis',(0.,0.70710678118655,-0.707106781186545));
#22819=DIRECTION('',(1.,0.,0.));
#22820=DIRECTION('center_axis',(0.,0.,1.));
#22821=DIRECTION('ref_axis',(1.,0.,0.));
#22822=DIRECTION('',(1.,0.,0.));
#22823=DIRECTION('',(0.,-1.,0.));
#22824=DIRECTION('center_axis',(0.,1.,0.));
#22825=DIRECTION('ref_axis',(-0.796497710072375,0.,0.604641544925142));
#22826=DIRECTION('center_axis',(0.,1.,0.));
#22827=DIRECTION('ref_axis',(-1.,0.,0.));
#22828=DIRECTION('',(0.,1.,0.));
#22829=DIRECTION('center_axis',(0.,-1.,0.));
#22830=DIRECTION('ref_axis',(-0.268817204301075,0.,0.963191211894998));
#22831=DIRECTION('',(0.,-1.,0.));
#22832=DIRECTION('center_axis',(0.,0.,1.));
#22833=DIRECTION('ref_axis',(1.,0.,0.));
#22834=DIRECTION('center_axis',(0.,0.,1.));
#22835=DIRECTION('ref_axis',(-0.707106781186544,0.707106781186551,0.));
#22836=DIRECTION('center_axis',(0.,0.,1.));
#22837=DIRECTION('ref_axis',(1.,0.,0.));
#22838=DIRECTION('center_axis',(0.,0.,1.));
#22839=DIRECTION('ref_axis',(-0.707106781186544,-0.707106781186551,0.));
#22840=DIRECTION('center_axis',(-0.963191211894998,0.,-0.268817204301074));
#22841=DIRECTION('ref_axis',(0.268817204301074,0.,-0.963191211894998));
#22842=DIRECTION('center_axis',(0.,0.,1.));
#22843=DIRECTION('ref_axis',(-0.707106781186542,0.707106781186553,0.));
#22844=DIRECTION('',(0.,0.,-1.));
#22845=DIRECTION('center_axis',(0.,0.,-1.));
#22846=DIRECTION('ref_axis',(-0.707106781186544,0.707106781186551,0.));
#22847=DIRECTION('',(0.,0.,1.));
#22848=DIRECTION('center_axis',(0.,1.,0.));
#22849=DIRECTION('ref_axis',(1.,0.,0.));
#22850=DIRECTION('center_axis',(0.,1.,0.));
#22851=DIRECTION('ref_axis',(0.707106781186547,0.,0.707106781186547));
#22852=DIRECTION('center_axis',(0.,1.,0.));
#22853=DIRECTION('ref_axis',(0.,0.,1.));
#22854=DIRECTION('center_axis',(0.,-1.,0.));
#22855=DIRECTION('ref_axis',(1.,0.,0.));
#22856=DIRECTION('center_axis',(-1.,0.,0.));
#22857=DIRECTION('ref_axis',(0.,0.,-1.));
#22858=DIRECTION('center_axis',(0.,1.,0.));
#22859=DIRECTION('ref_axis',(1.,0.,0.));
#22860=DIRECTION('center_axis',(0.,1.,0.));
#22861=DIRECTION('ref_axis',(1.,0.,0.));
#22862=DIRECTION('center_axis',(0.,1.,0.));
#22863=DIRECTION('ref_axis',(1.,0.,0.));
#22864=DIRECTION('',(0.707106781186548,0.,-0.707106781186547));
#22865=DIRECTION('',(0.,0.,-1.));
#22866=DIRECTION('',(1.,0.,0.));
#22867=DIRECTION('',(0.,0.,-1.));
#22868=DIRECTION('',(-1.,0.,0.));
#22869=DIRECTION('',(0.,0.,-1.));
#22870=DIRECTION('',(1.,0.,0.));
#22871=DIRECTION('',(0.707106781186547,0.,0.707106781186548));
#22872=DIRECTION('',(0.,0.,1.));
#22873=DIRECTION('',(-0.66436383882992,0.,0.74740931868366));
#22874=DIRECTION('',(-1.,0.,0.));
#22875=DIRECTION('',(-0.66436383882992,0.,-0.74740931868366));
#22876=DIRECTION('',(0.,0.,-1.));
#22877=DIRECTION('',(0.707106781186547,0.,-0.707106781186548));
#22878=DIRECTION('',(1.,0.,0.));
#22879=DIRECTION('',(0.,0.,1.));
#22880=DIRECTION('',(-1.,0.,0.));
#22881=DIRECTION('',(0.,0.,1.));
#22882=DIRECTION('',(1.,0.,0.));
#22883=DIRECTION('',(0.,0.,1.));
#22884=DIRECTION('',(0.707106781186548,0.,0.707106781186547));
#22885=DIRECTION('',(0.,0.,1.));
#22886=DIRECTION('center_axis',(0.,-1.,0.));
#22887=DIRECTION('ref_axis',(6.46422633350345E-16,0.,-1.));
#22888=DIRECTION('',(0.,0.,-1.));
#22889=DIRECTION('center_axis',(0.,-1.,0.));
#22890=DIRECTION('ref_axis',(1.,0.,0.));
#22891=DIRECTION('',(0.,0.,1.));
#22892=DIRECTION('center_axis',(0.,-1.,0.));
#22893=DIRECTION('ref_axis',(1.61616654811585E-15,0.,-1.));
#22894=DIRECTION('',(0.,0.,-1.));
#22895=DIRECTION('center_axis',(0.,-1.,0.));
#22896=DIRECTION('ref_axis',(1.49370186820111E-15,0.,1.));
#22897=DIRECTION('',(0.,0.,1.));
#22898=DIRECTION('center_axis',(0.,-1.,0.));
#22899=DIRECTION('ref_axis',(0.826936230559386,0.,-0.562295714538386));
#22900=DIRECTION('',(1.,0.,0.));
#22901=DIRECTION('center_axis',(0.,-1.,0.));
#22902=DIRECTION('ref_axis',(-0.826936230559385,0.,-0.562295714538387));
#22903=DIRECTION('',(0.,0.,-1.));
#22904=DIRECTION('center_axis',(0.,-1.,0.));
#22905=DIRECTION('ref_axis',(-0.707106781186547,0.,0.707106781186547));
#22906=DIRECTION('',(-1.,0.,0.));
#22907=DIRECTION('center_axis',(0.,-1.,0.));
#22908=DIRECTION('ref_axis',(0.707106781186547,0.,0.707106781186547));
#22909=DIRECTION('center_axis',(0.,-1.,0.));
#22910=DIRECTION('ref_axis',(1.,0.,0.));
#22911=DIRECTION('center_axis',(0.,-1.,0.));
#22912=DIRECTION('ref_axis',(-0.826936230559386,0.,0.562295714538386));
#22913=DIRECTION('',(-1.,0.,0.));
#22914=DIRECTION('center_axis',(0.,-1.,0.));
#22915=DIRECTION('ref_axis',(0.826936230559385,0.,0.562295714538387));
#22916=DIRECTION('',(0.,0.,1.));
#22917=DIRECTION('center_axis',(0.,-1.,0.));
#22918=DIRECTION('ref_axis',(0.707106781186547,0.,-0.707106781186548));
#22919=DIRECTION('',(1.,0.,0.));
#22920=DIRECTION('center_axis',(0.,-1.,0.));
#22921=DIRECTION('ref_axis',(-0.604641544925142,0.,-0.796497710072375));
#22922=DIRECTION('',(0.,0.,-1.));
#22923=DIRECTION('center_axis',(0.,-1.,0.));
#22924=DIRECTION('ref_axis',(1.,0.,0.));
#22925=DIRECTION('center_axis',(0.,1.,0.));
#22926=DIRECTION('ref_axis',(1.,0.,0.));
#22927=DIRECTION('',(0.,1.,0.));
#22928=DIRECTION('center_axis',(0.,-1.,0.));
#22929=DIRECTION('ref_axis',(1.,0.,0.));
#22930=DIRECTION('center_axis',(0.,-1.,0.));
#22931=DIRECTION('ref_axis',(1.,0.,0.));
#22932=DIRECTION('center_axis',(0.,1.,0.));
#22933=DIRECTION('ref_axis',(0.,0.,1.));
#22934=DIRECTION('center_axis',(-1.,0.,0.));
#22935=DIRECTION('ref_axis',(0.,0.,-1.));
#22936=DIRECTION('center_axis',(0.,1.,0.));
#22937=DIRECTION('ref_axis',(1.,0.,0.));
#22938=DIRECTION('center_axis',(0.,1.,0.));
#22939=DIRECTION('ref_axis',(1.,0.,0.));
#22940=DIRECTION('center_axis',(0.,1.,0.));
#22941=DIRECTION('ref_axis',(1.,0.,0.));
#22942=DIRECTION('',(0.,1.,0.));
#22943=DIRECTION('center_axis',(0.,-1.,0.));
#22944=DIRECTION('ref_axis',(1.,0.,0.));
#22945=DIRECTION('center_axis',(0.,-1.,0.));
#22946=DIRECTION('ref_axis',(1.,0.,0.));
#22947=DIRECTION('center_axis',(0.,1.,0.));
#22948=DIRECTION('ref_axis',(0.,0.,1.));
#22949=DIRECTION('center_axis',(-1.,0.,0.));
#22950=DIRECTION('ref_axis',(0.,0.,-1.));
#22951=DIRECTION('center_axis',(0.,0.,-1.));
#22952=DIRECTION('ref_axis',(-0.707106781186544,-0.707106781186551,0.));
#22953=DIRECTION('center_axis',(0.,0.,-1.));
#22954=DIRECTION('ref_axis',(0.,-1.,0.));
#22955=DIRECTION('',(0.,0.,-1.));
#22956=DIRECTION('center_axis',(0.,0.,1.));
#22957=DIRECTION('ref_axis',(-1.,0.,0.));
#22958=DIRECTION('center_axis',(0.,1.,0.));
#22959=DIRECTION('ref_axis',(1.65389215948551E-15,0.,-1.));
#22960=DIRECTION('center_axis',(0.,0.,-1.));
#22961=DIRECTION('ref_axis',(1.,0.,0.));
#22962=DIRECTION('center_axis',(0.,1.,0.));
#22963=DIRECTION('ref_axis',(1.61616654811585E-15,0.,-1.));
#22964=DIRECTION('center_axis',(0.,0.,1.));
#22965=DIRECTION('ref_axis',(0.707106781186544,-0.707106781186551,0.));
#22966=DIRECTION('center_axis',(0.,0.,-1.));
#22967=DIRECTION('ref_axis',(1.,0.,0.));
#22968=DIRECTION('',(0.,0.,1.));
#22969=DIRECTION('center_axis',(0.,1.,0.));
#22970=DIRECTION('ref_axis',(0.,0.,1.));
#22971=DIRECTION('center_axis',(0.,1.,0.));
#22972=DIRECTION('ref_axis',(1.49370186820111E-15,0.,1.));
#22973=DIRECTION('center_axis',(0.,1.,0.));
#22974=DIRECTION('ref_axis',(1.,0.,1.55493420815848E-15));
#22975=DIRECTION('',(0.,1.,0.));
#22976=DIRECTION('center_axis',(0.,-1.,0.));
#22977=DIRECTION('ref_axis',(1.61616654811585E-15,0.,-1.));
#22978=DIRECTION('',(0.,1.,0.));
#22979=DIRECTION('center_axis',(1.,0.,0.));
#22980=DIRECTION('ref_axis',(0.,0.,-1.));
#22981=DIRECTION('',(0.,1.,0.));
#22982=DIRECTION('',(0.,0.,1.));
#22983=DIRECTION('center_axis',(0.,0.,-1.));
#22984=DIRECTION('ref_axis',(-0.707106781186542,-0.707106781186553,0.));
#22985=DIRECTION('',(0.,0.,-1.));
#22986=DIRECTION('center_axis',(0.,0.,1.));
#22987=DIRECTION('ref_axis',(-1.,0.,0.));
#22988=DIRECTION('center_axis',(0.,1.,0.));
#22989=DIRECTION('ref_axis',(0.,0.,1.));
#22990=DIRECTION('center_axis',(0.321470784124453,-0.846950546350569,0.423475273175284));
#22991=DIRECTION('ref_axis',(-0.512101486820598,-0.531671676917694,-0.674594170712778));
#22992=DIRECTION('center_axis',(-1.,0.,0.));
#22993=DIRECTION('ref_axis',(0.,0.,-1.));
#22994=DIRECTION('center_axis',(0.268817204301076,0.,-0.963191211894997));
#22995=DIRECTION('ref_axis',(0.963191211894997,0.,0.268817204301076));
#22996=DIRECTION('center_axis',(0.,-1.,0.));
#22997=DIRECTION('ref_axis',(-0.60464154492514,0.,-0.796497710072376));
#22998=DIRECTION('center_axis',(1.,0.,0.));
#22999=DIRECTION('ref_axis',(0.,-0.70710678118655,-0.707106781186545));
#23000=DIRECTION('center_axis',(0.,0.,1.));
#23001=DIRECTION('ref_axis',(1.,0.,0.));
#23002=DIRECTION('center_axis',(0.,-1.,0.));
#23003=DIRECTION('ref_axis',(-0.796497710072374,0.,-0.604641544925144));
#23004=DIRECTION('center_axis',(-0.963191211894998,0.,0.268817204301074));
#23005=DIRECTION('ref_axis',(0.268817204301074,0.,0.963191211894998));
#23006=DIRECTION('center_axis',(1.,0.,0.));
#23007=DIRECTION('ref_axis',(0.,0.,-1.));
#23008=DIRECTION('',(0.,1.,0.));
#23009=DIRECTION('center_axis',(0.,1.,0.));
#23010=DIRECTION('ref_axis',(-0.60464154492514,0.,-0.796497710072376));
#23011=DIRECTION('',(0.,1.,0.));
#23012=DIRECTION('center_axis',(0.,-1.,0.));
#23013=DIRECTION('ref_axis',(-0.963191211894997,0.,-0.268817204301076));
#23014=DIRECTION('center_axis',(0.,1.,0.));
#23015=DIRECTION('ref_axis',(0.,0.,1.));
#23016=DIRECTION('center_axis',(0.963191211894997,0.,-0.268817204301076));
#23017=DIRECTION('ref_axis',(0.,-1.,0.));
#23018=DIRECTION('center_axis',(0.,1.,0.));
#23019=DIRECTION('ref_axis',(-0.707106781186547,0.,0.707106781186547));
#23020=DIRECTION('center_axis',(0.707106781186548,0.,-0.707106781186547));
#23021=DIRECTION('ref_axis',(0.500000000000001,-0.707106781186545,0.500000000000002));
#23022=DIRECTION('center_axis',(-0.382683432365091,0.,0.923879532511286));
#23023=DIRECTION('ref_axis',(0.923879532511286,6.94492722742783E-16,0.382683432365091));
#23024=DIRECTION('center_axis',(-0.707106781186548,0.,0.707106781186547));
#23025=DIRECTION('ref_axis',(0.,-1.,0.));
#23026=DIRECTION('',(-0.707106781186548,0.,0.707106781186547));
#23027=DIRECTION('center_axis',(0.,0.,1.));
#23028=DIRECTION('ref_axis',(1.,0.,0.));
#23029=DIRECTION('center_axis',(0.,0.,1.));
#23030=DIRECTION('ref_axis',(0.707106781186551,-0.707106781186544,0.));
#23031=DIRECTION('center_axis',(0.,-1.,0.));
#23032=DIRECTION('ref_axis',(0.923879532511287,0.,0.382683432365089));
#23033=DIRECTION('center_axis',(0.,0.,-1.));
#23034=DIRECTION('ref_axis',(0.70710678118655,-0.707106781186545,0.));
#23035=DIRECTION('center_axis',(0.,0.,1.));
#23036=DIRECTION('ref_axis',(0.,-1.,0.));
#23037=DIRECTION('',(0.,0.,1.));
#23038=DIRECTION('center_axis',(0.,0.,1.));
#23039=DIRECTION('ref_axis',(1.,0.,0.));
#23040=DIRECTION('center_axis',(0.,-1.,0.));
#23041=DIRECTION('ref_axis',(1.,0.,0.));
#23042=DIRECTION('center_axis',(2.96059473233375E-14,0.,-1.));
#23043=DIRECTION('ref_axis',(0.,-1.,0.));
#23044=DIRECTION('center_axis',(0.664363838829916,-4.91728020398219E-15,
0.747409318683663));
#23045=DIRECTION('ref_axis',(0.747409318683663,2.66054456061107E-31,-0.664363838829916));
#23046=DIRECTION('center_axis',(0.,0.,1.));
#23047=DIRECTION('ref_axis',(1.,0.,0.));
#23048=DIRECTION('center_axis',(0.,0.,1.));
#23049=DIRECTION('ref_axis',(-7.40148683083437E-15,-1.,0.));
#23050=DIRECTION('center_axis',(0.,-1.,0.));
#23051=DIRECTION('ref_axis',(0.923879532511288,0.,0.382683432365087));
#23052=DIRECTION('center_axis',(0.707106781186547,0.,-0.707106781186548));
#23053=DIRECTION('ref_axis',(0.500000000000006,-0.70710678118654,0.500000000000005));
#23054=DIRECTION('center_axis',(0.,0.,-1.));
#23055=DIRECTION('ref_axis',(0.707106781186547,-0.707106781186547,0.));
#23056=DIRECTION('',(0.,0.,1.));
#23057=DIRECTION('center_axis',(-0.196897064909128,-0.876918033036229,0.438459016518126));
#23058=DIRECTION('ref_axis',(0.359234778961065,-0.480639951872367,-0.799959755393309));
#23059=DIRECTION('center_axis',(0.,-1.,0.));
#23060=DIRECTION('ref_axis',(0.747409318683659,0.,-0.664363838829921));
#23061=DIRECTION('center_axis',(-0.664363838829928,0.,-0.747409318683652));
#23062=DIRECTION('ref_axis',(0.,-1.,0.));
#23063=DIRECTION('center_axis',(1.,7.40148683083437E-15,0.));
#23064=DIRECTION('ref_axis',(0.,0.,-1.));
#23065=DIRECTION('center_axis',(-0.66436383882992,0.,-0.74740931868366));
#23066=DIRECTION('ref_axis',(0.528498197563231,-0.70710678118655,-0.469776175611761));
#23067=DIRECTION('',(0.66436383882992,0.,0.74740931868366));
#23068=DIRECTION('center_axis',(0.196897064909139,-0.876918033036233,0.438459016518113));
#23069=DIRECTION('ref_axis',(-0.359234778961077,-0.48063995187236,-0.799959755393308));
#23070=DIRECTION('center_axis',(0.,-1.,0.));
#23071=DIRECTION('ref_axis',(0.,0.,-1.));
#23072=DIRECTION('center_axis',(-1.,0.,0.));
#23073=DIRECTION('ref_axis',(0.,-1.,0.));
#23074=DIRECTION('center_axis',(0.664363838829921,0.,-0.747409318683659));
#23075=DIRECTION('ref_axis',(-0.747409318683659,0.,-0.664363838829921));
#23076=DIRECTION('center_axis',(-1.,0.,0.));
#23077=DIRECTION('ref_axis',(0.,-0.707106781186542,-0.707106781186553));
#23078=DIRECTION('',(1.,0.,0.));
#23079=DIRECTION('center_axis',(-0.66436383882992,0.,0.74740931868366));
#23080=DIRECTION('ref_axis',(-0.528498197563231,-0.70710678118655,-0.469776175611761));
#23081=DIRECTION('center_axis',(0.664363838829924,0.,-0.747409318683656));
#23082=DIRECTION('ref_axis',(0.,-1.,0.));
#23083=DIRECTION('',(0.66436383882992,0.,-0.74740931868366));
#23084=DIRECTION('center_axis',(0.,0.,1.));
#23085=DIRECTION('ref_axis',(1.,0.,0.));
#23086=DIRECTION('center_axis',(0.,0.,-1.));
#23087=DIRECTION('ref_axis',(-0.707106781186547,-0.707106781186547,0.));
#23088=DIRECTION('center_axis',(0.,-1.,0.));
#23089=DIRECTION('ref_axis',(-0.934721701546419,0.,-0.355380557512882));
#23090=DIRECTION('center_axis',(0.,1.,0.));
#23091=DIRECTION('ref_axis',(-0.40965605156648,0.,-0.912240055804919));
#23092=DIRECTION('center_axis',(0.,-1.,0.));
#23093=DIRECTION('ref_axis',(-0.747409318683659,0.,-0.664363838829921));
#23094=DIRECTION('',(0.,-1.,0.));
#23095=DIRECTION('',(0.,1.,0.));
#23096=DIRECTION('center_axis',(-0.196897064909128,-0.876918033036235,-0.438459016518114));
#23097=DIRECTION('ref_axis',(-0.359234778961066,0.480639951872362,-0.799959755393312));
#23098=DIRECTION('center_axis',(0.66436383882992,0.,-0.74740931868366));
#23099=DIRECTION('ref_axis',(-0.528498197563228,0.707106781186555,-0.469776175611758));
#23100=DIRECTION('center_axis',(-1.,0.,0.));
#23101=DIRECTION('ref_axis',(0.,0.707106781186551,-0.707106781186544));
#23102=DIRECTION('center_axis',(0.,1.,0.));
#23103=DIRECTION('ref_axis',(0.40965605156648,0.,-0.912240055804919));
#23104=DIRECTION('center_axis',(0.,-1.,0.));
#23105=DIRECTION('ref_axis',(0.,0.,-1.));
#23106=DIRECTION('',(0.,-1.,0.));
#23107=DIRECTION('',(0.,1.,0.));
#23108=DIRECTION('center_axis',(0.196897064909128,-0.876918033036229,-0.438459016518126));
#23109=DIRECTION('ref_axis',(0.359234778961052,0.480639951872364,-0.799959755393317));
#23110=DIRECTION('center_axis',(1.,0.,0.));
#23111=DIRECTION('ref_axis',(0.,0.707106781186551,-0.707106781186544));
#23112=DIRECTION('center_axis',(-0.66436383882992,0.,-0.74740931868366));
#23113=DIRECTION('ref_axis',(0.528498197563224,0.70710678118656,-0.469776175611754));
#23114=DIRECTION('center_axis',(0.,1.,0.));
#23115=DIRECTION('ref_axis',(0.934721701546416,0.,-0.355380557512891));
#23116=DIRECTION('center_axis',(0.,-1.,0.));
#23117=DIRECTION('ref_axis',(0.747409318683655,0.,-0.664363838829925));
#23118=DIRECTION('',(0.,-1.,0.));
#23119=DIRECTION('',(0.,1.,0.));
#23120=DIRECTION('center_axis',(0.,0.,1.));
#23121=DIRECTION('ref_axis',(1.,0.,0.));
#23122=DIRECTION('center_axis',(0.66436383882992,0.,0.74740931868366));
#23123=DIRECTION('ref_axis',(0.528498197563228,0.707106781186555,-0.469776175611758));
#23124=DIRECTION('center_axis',(0.,0.,-1.));
#23125=DIRECTION('ref_axis',(0.707106781186544,0.707106781186551,0.));
#23126=DIRECTION('center_axis',(0.74740931868366,0.,-0.66436383882992));
#23127=DIRECTION('ref_axis',(-0.66436383882992,0.,-0.74740931868366));
#23128=DIRECTION('',(-0.66436383882992,0.,-0.74740931868366));
#23129=DIRECTION('center_axis',(0.,0.,-1.));
#23130=DIRECTION('ref_axis',(-1.,0.,0.));
#23131=DIRECTION('',(-1.,0.,0.));
#23132=DIRECTION('center_axis',(-1.,0.,0.));
#23133=DIRECTION('ref_axis',(0.,0.707106781186547,-0.707106781186547));
#23134=DIRECTION('',(1.,0.,0.));
#23135=DIRECTION('center_axis',(-0.66436383882992,0.,0.74740931868366));
#23136=DIRECTION('ref_axis',(-0.528498197563227,0.707106781186556,-0.469776175611757));
#23137=DIRECTION('',(-0.66436383882992,0.,0.74740931868366));
#23138=DIRECTION('center_axis',(-0.66436383882992,0.,0.74740931868366));
#23139=DIRECTION('ref_axis',(-0.528498197563228,0.707106781186555,-0.469776175611758));
#23140=DIRECTION('',(0.66436383882992,0.,-0.74740931868366));
#23141=DIRECTION('center_axis',(-0.74740931868366,0.,-0.66436383882992));
#23142=DIRECTION('ref_axis',(-0.66436383882992,0.,0.74740931868366));
#23143=DIRECTION('',(0.,-1.,0.));
#23144=DIRECTION('center_axis',(0.,0.,1.));
#23145=DIRECTION('ref_axis',(1.,0.,0.));
#23146=DIRECTION('center_axis',(0.,0.,1.));
#23147=DIRECTION('ref_axis',(1.,0.,0.));
#23148=DIRECTION('center_axis',(7.40148683083432E-15,-1.,-2.0656822580655E-15));
#23149=DIRECTION('ref_axis',(0.268817204301075,5.02404021851122E-31,0.963191211894998));
#23150=DIRECTION('center_axis',(0.963191211895,0.,-0.268817204301067));
#23151=DIRECTION('ref_axis',(0.,-1.,0.));
#23152=DIRECTION('center_axis',(0.,0.,1.));
#23153=DIRECTION('ref_axis',(1.,0.,0.));
#23154=DIRECTION('center_axis',(0.,1.,0.));
#23155=DIRECTION('ref_axis',(0.268817204301075,0.,0.963191211894998));
#23156=DIRECTION('center_axis',(0.,0.,1.));
#23157=DIRECTION('ref_axis',(0.707106781186544,0.707106781186551,0.));
#23158=DIRECTION('center_axis',(0.963191211894997,0.,-0.268817204301076));
#23159=DIRECTION('ref_axis',(-0.268817204301076,0.,-0.963191211894997));
#23160=DIRECTION('center_axis',(0.,-1.,0.));
#23161=DIRECTION('ref_axis',(0.796497710072375,0.,0.604641544925142));
#23162=DIRECTION('',(0.,-1.,0.));
#23163=DIRECTION('',(0.,1.,0.));
#23164=DIRECTION('center_axis',(0.,1.,0.));
#23165=DIRECTION('ref_axis',(0.,0.,1.));
#23166=DIRECTION('center_axis',(-0.268817204301074,1.78226176760406E-15,
0.963191211894998));
#23167=DIRECTION('ref_axis',(-0.963191211894998,7.01637702544147E-32,-0.268817204301074));
#23168=DIRECTION('center_axis',(0.,1.,0.));
#23169=DIRECTION('ref_axis',(-0.826936230559386,0.,0.562295714538386));
#23170=DIRECTION('center_axis',(0.321470784124458,-0.846950546350566,0.423475273175286));
#23171=DIRECTION('ref_axis',(-0.512101486820597,-0.531671676917699,-0.674594170712774));
#23172=DIRECTION('center_axis',(0.,-1.,0.));
#23173=DIRECTION('ref_axis',(-0.604641544925144,0.,-0.796497710072374));
#23174=DIRECTION('center_axis',(-1.,0.,0.));
#23175=DIRECTION('ref_axis',(0.,-0.70710678118655,-0.707106781186545));
#23176=DIRECTION('center_axis',(0.,0.,1.));
#23177=DIRECTION('ref_axis',(0.707106781186542,-0.707106781186553,0.));
#23178=DIRECTION('center_axis',(0.,0.,1.));
#23179=DIRECTION('ref_axis',(0.,-1.,0.));
#23180=DIRECTION('',(0.,0.,1.));
#23181=DIRECTION('center_axis',(0.,1.,0.));
#23182=DIRECTION('ref_axis',(-0.707106781186548,0.,-0.707106781186547));
#23183=DIRECTION('center_axis',(0.,1.,0.));
#23184=DIRECTION('ref_axis',(-0.604641544925142,0.,-0.796497710072375));
#23185=DIRECTION('center_axis',(-0.963191211894997,0.,-0.268817204301076));
#23186=DIRECTION('ref_axis',(0.268817204301076,0.,-0.963191211894997));
#23187=DIRECTION('center_axis',(-1.,0.,0.));
#23188=DIRECTION('ref_axis',(0.,-0.707106781186553,0.707106781186542));
#23189=DIRECTION('center_axis',(0.,1.,0.));
#23190=DIRECTION('ref_axis',(0.707106781186548,0.,-0.707106781186547));
#23191=DIRECTION('center_axis',(0.,0.,-1.));
#23192=DIRECTION('ref_axis',(-0.707106781186545,-0.70710678118655,0.));
#23193=DIRECTION('center_axis',(-0.321470784124458,-0.846950546350566,0.423475273175286));
#23194=DIRECTION('ref_axis',(0.512101486820597,-0.531671676917699,-0.674594170712774));
#23195=DIRECTION('center_axis',(-0.268817204301076,0.,-0.963191211894997));
#23196=DIRECTION('ref_axis',(0.963191211894997,0.,-0.268817204301076));
#23197=DIRECTION('center_axis',(1.,0.,0.));
#23198=DIRECTION('ref_axis',(0.,-0.70710678118655,-0.707106781186545));
#23199=DIRECTION('center_axis',(0.,-1.,0.));
#23200=DIRECTION('ref_axis',(0.60464154492514,0.,-0.796497710072376));
#23201=DIRECTION('center_axis',(0.,1.,0.));
#23202=DIRECTION('ref_axis',(0.,0.,1.));
#23203=DIRECTION('center_axis',(0.,0.,1.));
#23204=DIRECTION('ref_axis',(1.,0.,0.));
#23205=DIRECTION('center_axis',(0.,-1.,0.));
#23206=DIRECTION('ref_axis',(0.796497710072377,0.,-0.604641544925139));
#23207=DIRECTION('center_axis',(0.,-1.,0.));
#23208=DIRECTION('ref_axis',(-0.707106781186547,0.,0.707106781186548));
#23209=DIRECTION('center_axis',(0.,1.,0.));
#23210=DIRECTION('ref_axis',(-0.707106781186547,0.,0.707106781186547));
#23211=DIRECTION('center_axis',(0.268817204301076,0.,-0.963191211894997));
#23212=DIRECTION('ref_axis',(0.963191211894997,0.,0.268817204301076));
#23213=DIRECTION('center_axis',(0.,-1.,0.));
#23214=DIRECTION('ref_axis',(-0.707106781186547,0.,0.707106781186547));
#23215=DIRECTION('center_axis',(0.,0.,-1.));
#23216=DIRECTION('ref_axis',(0.707106781186542,0.707106781186553,0.));
#23217=DIRECTION('',(0.,0.,-1.));
#23218=DIRECTION('center_axis',(0.,0.,-1.));
#23219=DIRECTION('ref_axis',(0.707106781186544,0.707106781186551,0.));
#23220=DIRECTION('',(0.,0.,1.));
#23221=DIRECTION('center_axis',(-1.,0.,0.));
#23222=DIRECTION('ref_axis',(0.,0.,1.));
#23223=DIRECTION('',(0.,-1.,0.));
#23224=DIRECTION('center_axis',(0.,1.,0.));
#23225=DIRECTION('ref_axis',(0.796497710072378,0.,-0.604641544925139));
#23226=DIRECTION('',(0.,1.,0.));
#23227=DIRECTION('center_axis',(0.,-1.,0.));
#23228=DIRECTION('ref_axis',(0.268817204301081,0.,-0.963191211894996));
#23229=DIRECTION('center_axis',(0.,1.,0.));
#23230=DIRECTION('ref_axis',(-0.707106781186547,0.,-0.707106781186548));
#23231=DIRECTION('center_axis',(0.,-1.,0.));
#23232=DIRECTION('ref_axis',(0.60464154492514,0.,-0.796497710072376));
#23233=DIRECTION('',(0.,1.,0.));
#23234=DIRECTION('center_axis',(0.,1.,0.));
#23235=DIRECTION('ref_axis',(0.,0.,-1.));
#23236=DIRECTION('center_axis',(0.,1.,0.));
#23237=DIRECTION('ref_axis',(0.,0.,1.));
#23238=DIRECTION('center_axis',(-1.,0.,0.));
#23239=DIRECTION('ref_axis',(0.,0.,-1.));
#23240=DIRECTION('center_axis',(0.,1.,0.));
#23241=DIRECTION('ref_axis',(1.,0.,0.));
#23242=DIRECTION('center_axis',(0.,1.,0.));
#23243=DIRECTION('ref_axis',(1.,0.,0.));
#23244=DIRECTION('center_axis',(0.,1.,0.));
#23245=DIRECTION('ref_axis',(1.,0.,0.));
#23246=DIRECTION('',(0.,1.,0.));
#23247=DIRECTION('center_axis',(0.,-1.,0.));
#23248=DIRECTION('ref_axis',(1.,0.,0.));
#23249=DIRECTION('center_axis',(0.,-1.,0.));
#23250=DIRECTION('ref_axis',(1.,0.,0.));
#23251=DIRECTION('center_axis',(0.,0.,1.));
#23252=DIRECTION('ref_axis',(1.,0.,0.));
#23253=DIRECTION('center_axis',(0.,-1.,0.));
#23254=DIRECTION('ref_axis',(-1.,0.,0.));
#23255=DIRECTION('center_axis',(2.96059473233375E-14,0.,1.));
#23256=DIRECTION('ref_axis',(0.,-1.,0.));
#23257=DIRECTION('center_axis',(-0.707106781186544,3.14018491736755E-14,
-0.707106781186551));
#23258=DIRECTION('ref_axis',(-0.707106781186551,2.99807087075423E-31,0.707106781186544));
#23259=DIRECTION('center_axis',(0.,0.,1.));
#23260=DIRECTION('ref_axis',(-0.707106781186547,-0.707106781186547,0.));
#23261=DIRECTION('',(0.,0.,-1.));
#23262=DIRECTION('center_axis',(0.182143211721535,-0.879465224064607,-0.439732612032306));
#23263=DIRECTION('ref_axis',(-0.336556770590779,-0.475963149477974,0.812519920068741));
#23264=DIRECTION('center_axis',(0.,-1.,0.));
#23265=DIRECTION('ref_axis',(-0.707106781186548,0.,0.707106781186548));
#23266=DIRECTION('center_axis',(0.707106781186544,0.,0.707106781186551));
#23267=DIRECTION('ref_axis',(0.,-1.,0.));
#23268=DIRECTION('center_axis',(-1.,-7.40148683083437E-15,0.));
#23269=DIRECTION('ref_axis',(0.,0.,1.));
#23270=DIRECTION('center_axis',(0.707106781186547,0.,0.707106781186548));
#23271=DIRECTION('ref_axis',(-0.500000000000005,-0.70710678118654,0.500000000000005));
#23272=DIRECTION('',(-0.707106781186547,0.,-0.707106781186548));
#23273=DIRECTION('center_axis',(-0.408248290463862,-0.816496580927729,-0.408248290463859));
#23274=DIRECTION('ref_axis',(0.577350269189622,-0.577350269189622,0.577350269189634));
#23275=DIRECTION('center_axis',(0.,-1.,0.));
#23276=DIRECTION('ref_axis',(0.,0.,1.));
#23277=DIRECTION('center_axis',(1.,0.,0.));
#23278=DIRECTION('ref_axis',(0.,-1.,0.));
#23279=DIRECTION('center_axis',(0.,-1.48029736616687E-14,1.));
#23280=DIRECTION('ref_axis',(1.,0.,0.));
#23281=DIRECTION('center_axis',(1.,0.,0.));
#23282=DIRECTION('ref_axis',(0.,-0.707106781186542,0.707106781186553));
#23283=DIRECTION('',(-1.,0.,0.));
#23284=DIRECTION('center_axis',(-0.408248290463864,-0.816496580927728,0.408248290463858));
#23285=DIRECTION('ref_axis',(0.577350269189628,-0.577350269189628,-0.577350269189622));
#23286=DIRECTION('center_axis',(0.,-1.,0.));
#23287=DIRECTION('ref_axis',(1.,0.,0.));
#23288=DIRECTION('center_axis',(0.,0.,-1.));
#23289=DIRECTION('ref_axis',(0.,-1.,0.));
#23290=DIRECTION('center_axis',(1.,0.,0.));
#23291=DIRECTION('ref_axis',(0.,0.,-1.));
#23292=DIRECTION('center_axis',(0.,0.,-1.));
#23293=DIRECTION('ref_axis',(0.70710678118655,-0.707106781186545,0.));
#23294=DIRECTION('',(0.,0.,1.));
#23295=DIRECTION('center_axis',(-1.,0.,0.));
#23296=DIRECTION('ref_axis',(0.,-0.707106781186542,-0.707106781186553));
#23297=DIRECTION('',(1.,0.,0.));
#23298=DIRECTION('center_axis',(0.707106781186548,0.,0.707106781186548));
#23299=DIRECTION('ref_axis',(0.707106781186548,0.,-0.707106781186548));
#23300=DIRECTION('center_axis',(0.,0.,-1.));
#23301=DIRECTION('ref_axis',(0.70710678118655,-0.707106781186545,0.));
#23302=DIRECTION('center_axis',(-0.707106781186548,0.,0.707106781186548));
#23303=DIRECTION('ref_axis',(0.707106781186548,0.,0.707106781186548));
#23304=DIRECTION('',(0.,0.,1.));
#23305=DIRECTION('center_axis',(-0.816496580927727,-0.408248290463865,0.408248290463859));
#23306=DIRECTION('ref_axis',(0.577350269189626,-0.577350269189629,0.577350269189623));
#23307=DIRECTION('center_axis',(0.,-1.,0.));
#23308=DIRECTION('ref_axis',(0.,0.,1.));
#23309=DIRECTION('center_axis',(1.,0.,0.));
#23310=DIRECTION('ref_axis',(0.,-1.,0.));
#23311=DIRECTION('center_axis',(0.,7.40148683083437E-15,1.));
#23312=DIRECTION('ref_axis',(1.,0.,0.));
#23313=DIRECTION('center_axis',(1.,0.,0.));
#23314=DIRECTION('ref_axis',(0.,-0.707106781186547,0.707106781186547));
#23315=DIRECTION('',(-1.,0.,0.));
#23316=DIRECTION('center_axis',(0.,0.,-1.));
#23317=DIRECTION('ref_axis',(0.70710678118655,-0.707106781186545,0.));
#23318=DIRECTION('',(0.,0.,1.));
#23319=DIRECTION('center_axis',(0.,1.,0.));
#23320=DIRECTION('ref_axis',(0.707106781186545,0.,0.70710678118655));
#23321=DIRECTION('center_axis',(0.,-1.,0.));
#23322=DIRECTION('ref_axis',(1.,0.,0.));
#23323=DIRECTION('',(0.,-1.,0.));
#23324=DIRECTION('',(0.,1.,0.));
#23325=DIRECTION('center_axis',(-0.816496580927726,0.408248290463866,0.40824829046386));
#23326=DIRECTION('ref_axis',(0.577350269189626,0.577350269189629,0.577350269189623));
#23327=DIRECTION('center_axis',(0.,0.,1.));
#23328=DIRECTION('ref_axis',(0.707106781186544,0.707106781186551,0.));
#23329=DIRECTION('center_axis',(1.,0.,0.));
#23330=DIRECTION('ref_axis',(0.,0.707106781186551,0.707106781186544));
#23331=DIRECTION('center_axis',(0.,1.,0.));
#23332=DIRECTION('ref_axis',(0.707106781186545,0.,-0.70710678118655));
#23333=DIRECTION('center_axis',(0.,-1.,0.));
#23334=DIRECTION('ref_axis',(0.,0.,-1.));
#23335=DIRECTION('',(0.,-1.,0.));
#23336=DIRECTION('',(0.,1.,0.));
#23337=DIRECTION('center_axis',(0.408248290463864,-0.816496580927727,-0.408248290463861));
#23338=DIRECTION('ref_axis',(0.57735026918963,0.577350269189624,-0.577350269189624));
#23339=DIRECTION('center_axis',(1.,0.,0.));
#23340=DIRECTION('ref_axis',(0.,0.707106781186547,-0.707106781186547));
#23341=DIRECTION('center_axis',(0.,0.,-1.));
#23342=DIRECTION('ref_axis',(0.707106781186544,0.707106781186551,0.));
#23343=DIRECTION('center_axis',(0.,1.,0.));
#23344=DIRECTION('ref_axis',(0.707106781186555,0.,0.70710678118654));
#23345=DIRECTION('center_axis',(0.,-1.,0.));
#23346=DIRECTION('ref_axis',(1.,0.,0.));
#23347=DIRECTION('',(0.,-1.,0.));
#23348=DIRECTION('',(0.,1.,0.));
#23349=DIRECTION('center_axis',(0.408248290463861,-0.816496580927728,0.408248290463861));
#23350=DIRECTION('ref_axis',(0.577350269189622,0.577350269189622,0.577350269189634));
#23351=DIRECTION('center_axis',(0.,0.,1.));
#23352=DIRECTION('ref_axis',(0.707106781186544,0.707106781186551,0.));
#23353=DIRECTION('center_axis',(1.,0.,0.));
#23354=DIRECTION('ref_axis',(0.,0.707106781186551,0.707106781186544));
#23355=DIRECTION('center_axis',(0.,1.,0.));
#23356=DIRECTION('ref_axis',(-0.38268343236509,0.,0.923879532511287));
#23357=DIRECTION('center_axis',(0.,-1.,0.));
#23358=DIRECTION('ref_axis',(0.,0.,1.));
#23359=DIRECTION('',(0.,-1.,0.));
#23360=DIRECTION('',(0.,1.,0.));
#23361=DIRECTION('center_axis',(-0.182143211721524,-0.879465224064608,0.43973261203231));
#23362=DIRECTION('ref_axis',(-0.33655677059077,0.475963149477971,0.812519920068747));
#23363=DIRECTION('center_axis',(-1.,0.,0.));
#23364=DIRECTION('ref_axis',(0.,0.707106781186551,0.707106781186544));
#23365=DIRECTION('center_axis',(0.707106781186547,0.,0.707106781186548));
#23366=DIRECTION('ref_axis',(-0.500000000000004,0.707106781186542,0.500000000000004));
#23367=DIRECTION('center_axis',(0.,1.,0.));
#23368=DIRECTION('ref_axis',(-0.923879532511285,0.,0.382683432365094));
#23369=DIRECTION('center_axis',(0.,-1.,0.));
#23370=DIRECTION('ref_axis',(-0.707106781186548,0.,0.707106781186548));
#23371=DIRECTION('',(0.,-1.,0.));
#23372=DIRECTION('',(0.,1.,0.));
#23373=DIRECTION('center_axis',(0.,0.,1.));
#23374=DIRECTION('ref_axis',(1.,0.,0.));
#23375=DIRECTION('center_axis',(-0.707106781186547,0.,-0.707106781186548));
#23376=DIRECTION('ref_axis',(-0.500000000000006,0.70710678118654,0.500000000000005));
#23377=DIRECTION('center_axis',(0.,0.,1.));
#23378=DIRECTION('ref_axis',(-0.707106781186544,0.707106781186551,0.));
#23379=DIRECTION('center_axis',(0.,1.,0.));
#23380=DIRECTION('ref_axis',(-0.934721701546419,0.,-0.355380557512883));
#23381=DIRECTION('',(0.,1.,0.));
#23382=DIRECTION('center_axis',(0.,-1.,0.));
#23383=DIRECTION('ref_axis',(-1.,0.,0.));
#23384=DIRECTION('center_axis',(0.,0.,1.));
#23385=DIRECTION('ref_axis',(1.,0.,0.));
#23386=DIRECTION('center_axis',(0.,0.,-1.));
#23387=DIRECTION('ref_axis',(-0.707106781186544,0.707106781186551,0.));
#23388=DIRECTION('center_axis',(0.,0.,1.));
#23389=DIRECTION('ref_axis',(1.,0.,0.));
#23390=DIRECTION('',(1.,0.,0.));
#23391=DIRECTION('center_axis',(0.707106781186547,0.,0.707106781186548));
#23392=DIRECTION('ref_axis',(-0.500000000000002,0.707106781186545,0.500000000000001));
#23393=DIRECTION('',(-0.707106781186547,0.,-0.707106781186548));
#23394=DIRECTION('',(0.707106781186547,0.,0.707106781186548));
#23395=DIRECTION('center_axis',(1.,0.,0.));
#23396=DIRECTION('ref_axis',(0.,0.707106781186547,0.707106781186547));
#23397=DIRECTION('',(-1.,0.,0.));
#23398=DIRECTION('center_axis',(1.,0.,0.));
#23399=DIRECTION('ref_axis',(0.,0.,-1.));
#23400=DIRECTION('',(0.,0.,-1.));
#23401=DIRECTION('center_axis',(0.,0.,-1.));
#23402=DIRECTION('ref_axis',(0.707106781186545,0.70710678118655,0.));
#23403=DIRECTION('',(0.,0.,1.));
#23404=DIRECTION('center_axis',(-1.,0.,0.));
#23405=DIRECTION('ref_axis',(0.,0.707106781186547,-0.707106781186547));
#23406=DIRECTION('',(-1.,0.,0.));
#23407=DIRECTION('center_axis',(-0.707106781186548,0.,-0.707106781186548));
#23408=DIRECTION('ref_axis',(-0.707106781186548,0.,0.707106781186548));
#23409=DIRECTION('',(1.,0.,0.));
#23410=DIRECTION('center_axis',(0.,0.,-1.));
#23411=DIRECTION('ref_axis',(-1.,0.,0.));
#23412=DIRECTION('',(0.,1.,0.));
#23413=DIRECTION('center_axis',(1.,0.,0.));
#23414=DIRECTION('ref_axis',(0.,0.,-1.));
#23415=DIRECTION('',(0.,1.,0.));
#23416=DIRECTION('',(0.,0.,-1.));
#23417=DIRECTION('center_axis',(0.,0.,1.));
#23418=DIRECTION('ref_axis',(1.,0.,0.));
#23419=DIRECTION('',(1.,0.,0.));
#23420=DIRECTION('center_axis',(1.,0.,0.));
#23421=DIRECTION('ref_axis',(0.,0.707106781186553,0.707106781186542));
#23422=DIRECTION('',(-1.,0.,0.));
#23423=DIRECTION('center_axis',(0.707106781186548,0.,-0.707106781186548));
#23424=DIRECTION('ref_axis',(-0.707106781186548,0.,-0.707106781186548));
#23425=DIRECTION('center_axis',(0.,0.,-1.));
#23426=DIRECTION('ref_axis',(0.707106781186545,0.70710678118655,0.));
#23427=DIRECTION('',(0.,0.,-1.));
#23428=DIRECTION('center_axis',(0.382683432365085,0.,-0.923879532511289));
#23429=DIRECTION('ref_axis',(0.923879532511289,1.06845034268121E-16,0.382683432365085));
#23430=DIRECTION('',(0.,0.,1.));
#23431=DIRECTION('center_axis',(1.,0.,0.));
#23432=DIRECTION('ref_axis',(0.,0.,-1.));
#23433=DIRECTION('',(0.,1.,0.));
#23434=DIRECTION('center_axis',(0.,-1.,0.));
#23435=DIRECTION('ref_axis',(0.,0.,-1.));
#23436=DIRECTION('center_axis',(0.,1.,0.));
#23437=DIRECTION('ref_axis',(1.,0.,0.));
#23438=DIRECTION('center_axis',(-1.,0.,0.));
#23439=DIRECTION('ref_axis',(0.,0.,1.));
#23440=DIRECTION('center_axis',(0.,1.,0.));
#23441=DIRECTION('ref_axis',(1.,0.,0.));
#23442=DIRECTION('',(-0.707106781186548,0.,0.707106781186547));
#23443=DIRECTION('',(0.,0.,1.));
#23444=DIRECTION('center_axis',(0.,1.,0.));
#23445=DIRECTION('ref_axis',(6.46422633350345E-16,0.,-1.));
#23446=DIRECTION('',(0.,0.,-1.));
#23447=DIRECTION('',(-0.707106781186548,0.,-0.707106781186547));
#23448=DIRECTION('',(0.,0.,-1.));
#23449=DIRECTION('',(-1.,0.,0.));
#23450=DIRECTION('',(0.,0.,-1.));
#23451=DIRECTION('',(1.,0.,0.));
#23452=DIRECTION('',(0.,0.,-1.));
#23453=DIRECTION('',(-1.,0.,0.));
#23454=DIRECTION('',(-0.707106781186547,0.,0.707106781186548));
#23455=DIRECTION('',(0.,0.,1.));
#23456=DIRECTION('',(0.66436383882992,0.,0.74740931868366));
#23457=DIRECTION('',(0.,0.,-1.));
#23458=DIRECTION('',(0.,0.,1.));
#23459=DIRECTION('center_axis',(0.,1.,0.));
#23460=DIRECTION('ref_axis',(-0.707106781186547,0.,0.707106781186547));
#23461=DIRECTION('',(0.,0.,1.));
#23462=DIRECTION('center_axis',(0.,1.,0.));
#23463=DIRECTION('ref_axis',(-0.707106781186547,0.,-0.707106781186548));
#23464=DIRECTION('',(-1.,0.,0.));
#23465=DIRECTION('center_axis',(0.,1.,0.));
#23466=DIRECTION('ref_axis',(0.707106781186547,0.,-0.707106781186547));
#23467=DIRECTION('',(0.,0.,-1.));
#23468=DIRECTION('center_axis',(0.,1.,0.));
#23469=DIRECTION('ref_axis',(1.49370186820111E-15,0.,1.));
#23470=DIRECTION('',(0.,0.,1.));
#23471=DIRECTION('center_axis',(0.,1.,0.));
#23472=DIRECTION('ref_axis',(1.61616654811585E-15,0.,-1.));
#23473=DIRECTION('center_axis',(0.,1.,0.));
#23474=DIRECTION('ref_axis',(1.,0.,0.));
#23475=DIRECTION('',(1.,0.,0.));
#23476=DIRECTION('center_axis',(0.,1.,0.));
#23477=DIRECTION('ref_axis',(1.,0.,0.));
#23478=DIRECTION('center_axis',(0.,1.,0.));
#23479=DIRECTION('ref_axis',(1.,0.,0.));
#23480=DIRECTION('center_axis',(0.321470784124458,-0.846950546350566,-0.423475273175286));
#23481=DIRECTION('ref_axis',(0.512101486820597,0.531671676917699,-0.674594170712774));
#23482=DIRECTION('center_axis',(1.,0.,0.));
#23483=DIRECTION('ref_axis',(0.,1.,0.));
#23484=DIRECTION('center_axis',(-1.,0.,0.));
#23485=DIRECTION('ref_axis',(0.,0.70710678118655,-0.707106781186545));
#23486=DIRECTION('center_axis',(1.,0.,0.));
#23487=DIRECTION('ref_axis',(0.,0.,-1.));
#23488=DIRECTION('',(-1.,0.,0.));
#23489=DIRECTION('center_axis',(1.,0.,0.));
#23490=DIRECTION('ref_axis',(0.,-0.70710678118655,-0.707106781186545));
#23491=DIRECTION('',(1.,0.,0.));
#23492=DIRECTION('center_axis',(0.,1.,0.));
#23493=DIRECTION('ref_axis',(-0.604641544925143,0.,-0.796497710072374));
#23494=DIRECTION('',(0.,1.,0.));
#23495=DIRECTION('center_axis',(0.,-1.,0.));
#23496=DIRECTION('ref_axis',(-0.963191211894997,0.,-0.268817204301076));
#23497=DIRECTION('',(0.,-1.,0.));
#23498=DIRECTION('center_axis',(-0.321470784124459,-0.846950546350567,-0.423475273175284));
#23499=DIRECTION('ref_axis',(-0.512101486820603,0.531671676917699,-0.67459417071277));
#23500=DIRECTION('center_axis',(0.,0.,1.));
#23501=DIRECTION('ref_axis',(1.,0.,0.));
#23502=DIRECTION('center_axis',(0.,1.,0.));
#23503=DIRECTION('ref_axis',(-0.707106781186547,0.,0.707106781186548));
#23504=DIRECTION('center_axis',(0.,0.,1.));
#23505=DIRECTION('ref_axis',(1.,0.,0.));
#23506=DIRECTION('center_axis',(0.,0.,-1.));
#23507=DIRECTION('ref_axis',(0.707106781186545,0.70710678118655,0.));
#23508=DIRECTION('center_axis',(0.,0.,1.));
#23509=DIRECTION('ref_axis',(-0.707106781186542,0.707106781186553,0.));
#23510=DIRECTION('',(0.,0.,1.));
#23511=DIRECTION('center_axis',(-0.66436383882992,0.,-0.74740931868366));
#23512=DIRECTION('ref_axis',(0.528498197563227,0.707106781186556,-0.469776175611757));
#23513=DIRECTION('center_axis',(0.,0.,1.));
#23514=DIRECTION('ref_axis',(1.,0.,0.));
#23515=DIRECTION('center_axis',(0.,0.,1.));
#23516=DIRECTION('ref_axis',(1.,0.,0.));
#23517=DIRECTION('center_axis',(0.707106781186547,0.,-0.707106781186548));
#23518=DIRECTION('ref_axis',(0.500000000000006,0.70710678118654,0.500000000000005));
#23519=DIRECTION('center_axis',(0.,1.,0.));
#23520=DIRECTION('ref_axis',(0.923879532511288,0.,0.382683432365087));
#23521=DIRECTION('center_axis',(0.,0.,-1.));
#23522=DIRECTION('ref_axis',(0.707106781186542,0.707106781186553,0.));
#23523=DIRECTION('',(0.,0.,-1.));
#23524=DIRECTION('center_axis',(-0.707106781186548,0.,0.707106781186547));
#23525=DIRECTION('ref_axis',(0.707106781186547,0.,0.707106781186548));
#23526=DIRECTION('center_axis',(-1.,0.,0.));
#23527=DIRECTION('ref_axis',(0.,0.,1.));
#23528=DIRECTION('center_axis',(1.,0.,0.));
#23529=DIRECTION('ref_axis',(0.,0.,-1.));
#23530=DIRECTION('',(0.,1.,0.));
#23531=DIRECTION('center_axis',(0.,1.,0.));
#23532=DIRECTION('ref_axis',(0.923879532511291,0.,0.38268343236508));
#23533=DIRECTION('',(0.,-1.,0.));
#23534=DIRECTION('center_axis',(0.,0.,1.));
#23535=DIRECTION('ref_axis',(1.,0.,0.));
#23536=DIRECTION('center_axis',(7.40148683083437E-15,-1.,-2.06568225806552E-15));
#23537=DIRECTION('ref_axis',(0.268817204301075,-3.31042368671712E-30,0.963191211894998));
#23538=DIRECTION('center_axis',(0.,0.,1.));
#23539=DIRECTION('ref_axis',(1.,0.,0.));
#23540=DIRECTION('center_axis',(0.,0.,1.));
#23541=DIRECTION('ref_axis',(1.,0.,0.));
#23542=DIRECTION('center_axis',(0.,-1.,0.));
#23543=DIRECTION('ref_axis',(1.,0.,0.));
#23544=DIRECTION('center_axis',(0.,0.,-1.));
#23545=DIRECTION('ref_axis',(0.,-1.,0.));
#23546=DIRECTION('center_axis',(0.963191211894997,0.,0.268817204301076));
#23547=DIRECTION('ref_axis',(0.268817204301076,0.,-0.963191211894997));
#23548=DIRECTION('center_axis',(0.,0.,1.));
#23549=DIRECTION('ref_axis',(0.707106781186545,-0.70710678118655,0.));
#23550=DIRECTION('',(0.,0.,1.));
#23551=DIRECTION('center_axis',(0.321470784124458,-0.846950546350565,-0.423475273175289));
#23552=DIRECTION('ref_axis',(-0.512101486820596,-0.531671676917698,0.674594170712776));
#23553=DIRECTION('center_axis',(0.268817204301076,0.,0.963191211894997));
#23554=DIRECTION('ref_axis',(-0.963191211894997,0.,0.268817204301076));
#23555=DIRECTION('center_axis',(-1.,0.,0.));
#23556=DIRECTION('ref_axis',(0.,-0.707106781186551,0.707106781186544));
#23557=DIRECTION('center_axis',(0.,-1.,0.));
#23558=DIRECTION('ref_axis',(-0.604641544925141,0.,0.796497710072376));
#23559=DIRECTION('center_axis',(0.,1.,0.));
#23560=DIRECTION('ref_axis',(-0.707106781186548,0.,-0.707106781186547));
#23561=DIRECTION('center_axis',(0.,1.,0.));
#23562=DIRECTION('ref_axis',(-0.826936230559385,0.,-0.562295714538387));
#23563=DIRECTION('center_axis',(0.,1.,0.));
#23564=DIRECTION('ref_axis',(0.796497710072379,0.,-0.604641544925138));
#23565=DIRECTION('center_axis',(0.,-1.,0.));
#23566=DIRECTION('ref_axis',(0.268817204301076,0.,-0.963191211894997));
#23567=DIRECTION('',(0.,-1.,0.));
#23568=DIRECTION('',(0.,1.,0.));
#23569=DIRECTION('center_axis',(0.,0.,1.));
#23570=DIRECTION('ref_axis',(1.,0.,0.));
#23571=DIRECTION('center_axis',(0.963191211894997,0.,0.268817204301076));
#23572=DIRECTION('ref_axis',(-0.268817204301076,0.,0.963191211894997));
#23573=DIRECTION('center_axis',(0.,0.,-1.));
#23574=DIRECTION('ref_axis',(0.707106781186544,0.707106781186551,0.));
#23575=DIRECTION('center_axis',(0.,0.,1.));
#23576=DIRECTION('ref_axis',(1.,0.,0.));
#23577=DIRECTION('center_axis',(0.,1.,0.));
#23578=DIRECTION('ref_axis',(0.268817204301075,0.,0.963191211894998));
#23579=DIRECTION('center_axis',(0.,0.,1.));
#23580=DIRECTION('ref_axis',(0.707106781186544,0.707106781186551,0.));
#23581=DIRECTION('center_axis',(0.963191211894997,0.,-0.268817204301076));
#23582=DIRECTION('ref_axis',(-0.268817204301076,0.,-0.963191211894997));
#23583=DIRECTION('center_axis',(0.,-1.,0.));
#23584=DIRECTION('ref_axis',(0.796497710072376,0.,0.60464154492514));
#23585=DIRECTION('',(0.,-1.,0.));
#23586=DIRECTION('',(0.,1.,0.));
#23587=DIRECTION('center_axis',(-0.321470784124459,-0.846950546350567,-0.423475273175284));
#23588=DIRECTION('ref_axis',(-0.512101486820597,0.531671676917699,-0.674594170712774));
#23589=DIRECTION('center_axis',(0.268817204301076,0.,-0.963191211894997));
#23590=DIRECTION('ref_axis',(0.963191211894997,0.,0.268817204301076));
#23591=DIRECTION('center_axis',(0.,1.,0.));
#23592=DIRECTION('ref_axis',(-0.707106781186547,0.,0.707106781186547));
#23593=DIRECTION('center_axis',(0.,-1.,0.));
#23594=DIRECTION('ref_axis',(-0.707106781186547,0.,0.707106781186547));
#23595=DIRECTION('center_axis',(0.,-1.,0.));
#23596=DIRECTION('ref_axis',(-0.707106781186547,0.,0.707106781186548));
#23597=DIRECTION('center_axis',(0.,0.,1.));
#23598=DIRECTION('ref_axis',(1.,0.,0.));
#23599=DIRECTION('center_axis',(0.,1.,0.));
#23600=DIRECTION('ref_axis',(-0.268817204301076,0.,-0.963191211894997));
#23601=DIRECTION('center_axis',(-0.963191211894997,0.,0.268817204301077));
#23602=DIRECTION('ref_axis',(0.268817204301077,0.,0.963191211894997));
#23603=DIRECTION('center_axis',(0.,-1.,0.));
#23604=DIRECTION('ref_axis',(-0.796497710072374,0.,-0.604641544925143));
#23605=DIRECTION('',(0.,-1.,0.));
#23606=DIRECTION('center_axis',(0.,1.,0.));
#23607=DIRECTION('ref_axis',(0.707106781186548,0.,-0.707106781186547));
#23608=DIRECTION('center_axis',(0.,1.,0.));
#23609=DIRECTION('ref_axis',(0.826936230559386,0.,-0.562295714538385));
#23610=DIRECTION('center_axis',(0.268817204301074,0.,-0.963191211894998));
#23611=DIRECTION('ref_axis',(0.963191211894998,0.,0.268817204301074));
#23612=DIRECTION('center_axis',(-0.321470784124458,-0.846950546350565,-0.423475273175289));
#23613=DIRECTION('ref_axis',(0.512101486820605,-0.531671676917701,0.674594170712767));
#23614=DIRECTION('center_axis',(0.,-1.,0.));
#23615=DIRECTION('ref_axis',(0.604641544925144,0.,0.796497710072374));
#23616=DIRECTION('center_axis',(1.,0.,0.));
#23617=DIRECTION('ref_axis',(0.,-0.707106781186551,0.707106781186544));
#23618=DIRECTION('center_axis',(0.,-1.,0.));
#23619=DIRECTION('ref_axis',(0.,0.,-1.));
#23620=DIRECTION('center_axis',(-0.268817204301076,0.,0.963191211894997));
#23621=DIRECTION('ref_axis',(-0.963191211894997,0.,-0.268817204301076));
#23622=DIRECTION('center_axis',(0.,-1.,0.));
#23623=DIRECTION('ref_axis',(0.707106781186547,0.,-0.707106781186547));
#23624=DIRECTION('center_axis',(-0.321470784124458,-0.846950546350565,0.423475273175289));
#23625=DIRECTION('ref_axis',(-0.512101486820596,0.531671676917698,0.674594170712776));
#23626=DIRECTION('center_axis',(0.,1.,0.));
#23627=DIRECTION('ref_axis',(-0.963191211894998,0.,0.268817204301075));
#23628=DIRECTION('center_axis',(-1.,0.,0.));
#23629=DIRECTION('ref_axis',(0.,0.707106781186551,0.707106781186544));
#23630=DIRECTION('center_axis',(0.268817204301076,0.,0.963191211894997));
#23631=DIRECTION('ref_axis',(0.963191211894997,0.,-0.268817204301076));
#23632=DIRECTION('center_axis',(0.,-1.,0.));
#23633=DIRECTION('ref_axis',(-0.60464154492514,0.,0.796497710072376));
#23634=DIRECTION('',(0.,1.,0.));
#23635=DIRECTION('',(0.,-1.,0.));
#23636=DIRECTION('center_axis',(-1.,0.,0.));
#23637=DIRECTION('ref_axis',(0.,-0.707106781186553,0.707106781186542));
#23638=DIRECTION('',(-1.,0.,0.));
#23639=DIRECTION('center_axis',(0.,1.,0.));
#23640=DIRECTION('ref_axis',(0.604641544925143,0.,0.796497710072374));
#23641=DIRECTION('',(0.,1.,0.));
#23642=DIRECTION('center_axis',(0.,-1.,0.));
#23643=DIRECTION('ref_axis',(0.963191211894998,0.,0.268817204301074));
#23644=DIRECTION('',(0.,-1.,0.));
#23645=DIRECTION('center_axis',(0.32147078412446,-0.84695054635057,0.423475273175279));
#23646=DIRECTION('ref_axis',(0.512101486820602,0.531671676917693,0.674594170712776));
#23647=DIRECTION('center_axis',(1.,0.,0.));
#23648=DIRECTION('ref_axis',(0.,0.707106781186551,0.707106781186544));
#23649=DIRECTION('center_axis',(0.,0.,-1.));
#23650=DIRECTION('ref_axis',(-1.,0.,0.));
#23651=DIRECTION('',(1.,0.,0.));
#23652=DIRECTION('center_axis',(0.,1.,0.));
#23653=DIRECTION('ref_axis',(1.,0.,0.));
#23654=DIRECTION('center_axis',(0.707106781186548,0.,-0.707106781186547));
#23655=DIRECTION('ref_axis',(0.499999999999998,0.707106781186551,0.499999999999998));
#23656=DIRECTION('center_axis',(-0.707106781186548,0.,0.707106781186548));
#23657=DIRECTION('ref_axis',(0.707106781186547,0.,0.707106781186547));
#23658=DIRECTION('',(0.707106781186548,0.,-0.707106781186547));
#23659=DIRECTION('center_axis',(0.,0.,1.));
#23660=DIRECTION('ref_axis',(1.,0.,0.));
#23661=DIRECTION('center_axis',(0.,-1.,0.));
#23662=DIRECTION('ref_axis',(-1.,0.,0.));
#23663=DIRECTION('center_axis',(-3.70074341541718E-15,0.,1.));
#23664=DIRECTION('ref_axis',(0.,-1.,0.));
#23665=DIRECTION('center_axis',(-0.707106781186548,-2.61682076447296E-15,
-0.707106781186548));
#23666=DIRECTION('ref_axis',(-0.707106781186547,-1.53081335547773E-32,0.707106781186547));
#23667=DIRECTION('center_axis',(0.,1.,0.));
#23668=DIRECTION('ref_axis',(1.01064309961486E-15,0.,-1.));
#23669=DIRECTION('center_axis',(0.,0.,-1.));
#23670=DIRECTION('ref_axis',(0.,-1.,0.));
#23671=DIRECTION('center_axis',(0.,1.,0.));
#23672=DIRECTION('ref_axis',(6.46422633350345E-16,0.,-1.));
#23673=DIRECTION('center_axis',(0.,0.,1.));
#23674=DIRECTION('ref_axis',(-0.70710678118655,-0.707106781186545,0.));
#23675=DIRECTION('',(0.,0.,-1.));
#23676=DIRECTION('center_axis',(0.707106781186548,0.,0.707106781186547));
#23677=DIRECTION('ref_axis',(-0.500000000000001,-0.707106781186545,0.500000000000002));
#23678=DIRECTION('',(-0.707106781186548,0.,-0.707106781186547));
#23679=DIRECTION('center_axis',(-0.382683432365088,0.,-0.923879532511288));
#23680=DIRECTION('ref_axis',(-0.923879532511288,0.,0.382683432365088));
#23681=DIRECTION('center_axis',(0.408248290463864,-0.816496580927728,-0.408248290463858));
#23682=DIRECTION('ref_axis',(-0.577350269189628,-0.577350269189628,0.577350269189622));
#23683=DIRECTION('center_axis',(0.,-1.,0.));
#23684=DIRECTION('ref_axis',(-1.,0.,0.));
#23685=DIRECTION('center_axis',(0.,0.,1.));
#23686=DIRECTION('ref_axis',(0.,-1.,0.));
#23687=DIRECTION('center_axis',(-1.,0.,0.));
#23688=DIRECTION('ref_axis',(0.,0.,1.));
#23689=DIRECTION('center_axis',(0.,0.,1.));
#23690=DIRECTION('ref_axis',(-0.70710678118655,-0.707106781186545,0.));
#23691=DIRECTION('',(0.,0.,-1.));
#23692=DIRECTION('center_axis',(1.,0.,0.));
#23693=DIRECTION('ref_axis',(0.,-0.707106781186547,0.707106781186547));
#23694=DIRECTION('',(-1.,0.,0.));
#23695=DIRECTION('center_axis',(-0.707106781186548,0.,-0.707106781186548));
#23696=DIRECTION('ref_axis',(-0.707106781186548,0.,0.707106781186548));
#23697=DIRECTION('center_axis',(0.,0.,1.));
#23698=DIRECTION('ref_axis',(-0.70710678118655,-0.707106781186545,0.));
#23699=DIRECTION('center_axis',(0.707106781186548,0.,-0.707106781186548));
#23700=DIRECTION('ref_axis',(-0.707106781186548,0.,-0.707106781186548));
#23701=DIRECTION('',(0.,0.,-1.));
#23702=DIRECTION('center_axis',(0.408248290463864,-0.816496580927728,0.408248290463858));
#23703=DIRECTION('ref_axis',(-0.577350269189628,-0.577350269189628,-0.577350269189622));
#23704=DIRECTION('center_axis',(0.,-1.,0.));
#23705=DIRECTION('ref_axis',(0.,0.,-1.));
#23706=DIRECTION('center_axis',(-1.,0.,0.));
#23707=DIRECTION('ref_axis',(0.,-1.,0.));
#23708=DIRECTION('center_axis',(0.,0.,-1.));
#23709=DIRECTION('ref_axis',(-1.,0.,0.));
#23710=DIRECTION('center_axis',(-1.,0.,0.));
#23711=DIRECTION('ref_axis',(0.,-0.707106781186542,-0.707106781186553));
#23712=DIRECTION('',(1.,0.,0.));
#23713=DIRECTION('center_axis',(-0.816496580927727,0.408248290463865,-0.408248290463859));
#23714=DIRECTION('ref_axis',(-0.577350269189626,-0.577350269189629,0.577350269189623));
#23715=DIRECTION('center_axis',(0.,-1.,0.));
#23716=DIRECTION('ref_axis',(-1.,0.,0.));
#23717=DIRECTION('center_axis',(0.,0.,1.));
#23718=DIRECTION('ref_axis',(0.,-1.,0.));
#23719=DIRECTION('center_axis',(-1.,0.,0.));
#23720=DIRECTION('ref_axis',(0.,0.,1.));
#23721=DIRECTION('center_axis',(0.,0.,1.));
#23722=DIRECTION('ref_axis',(-0.70710678118655,-0.707106781186545,0.));
#23723=DIRECTION('',(0.,0.,-1.));
#23724=DIRECTION('center_axis',(-0.182143211721535,-0.879465224064607,-0.439732612032306));
#23725=DIRECTION('ref_axis',(0.33655677059079,-0.475963149477972,0.812519920068738));
#23726=DIRECTION('center_axis',(0.,-1.,0.));
#23727=DIRECTION('ref_axis',(0.,0.,1.));
#23728=DIRECTION('center_axis',(1.,0.,-7.40148683083442E-15));
#23729=DIRECTION('ref_axis',(0.,-1.,0.));
#23730=DIRECTION('center_axis',(-0.707106781186544,0.,0.707106781186551));
#23731=DIRECTION('ref_axis',(0.707106781186551,0.,0.707106781186544));
#23732=DIRECTION('center_axis',(1.,0.,0.));
#23733=DIRECTION('ref_axis',(0.,-0.707106781186542,0.707106781186553));
#23734=DIRECTION('',(-1.,0.,0.));
#23735=DIRECTION('center_axis',(0.707106781186547,0.,-0.707106781186548));
#23736=DIRECTION('ref_axis',(0.500000000000005,-0.70710678118654,0.500000000000005));
#23737=DIRECTION('',(-0.707106781186547,0.,0.707106781186548));
#23738=DIRECTION('center_axis',(0.,1.,0.));
#23739=DIRECTION('ref_axis',(0.38268343236509,0.,0.923879532511287));
#23740=DIRECTION('center_axis',(0.,-1.,0.));
#23741=DIRECTION('ref_axis',(0.707106781186551,0.,0.707106781186544));
#23742=DIRECTION('',(0.,-1.,0.));
#23743=DIRECTION('',(0.,1.,0.));
#23744=DIRECTION('center_axis',(0.707106781186547,0.,-0.707106781186548));
#23745=DIRECTION('ref_axis',(0.500000000000002,0.707106781186545,0.500000000000001));
#23746=DIRECTION('center_axis',(0.707106781186544,0.,-0.707106781186551));
#23747=DIRECTION('ref_axis',(0.,1.,0.));
#23748=DIRECTION('',(0.707106781186547,0.,-0.707106781186548));
#23749=DIRECTION('center_axis',(0.,1.,0.));
#23750=DIRECTION('ref_axis',(-0.707106781186545,0.,0.70710678118655));
#23751=DIRECTION('center_axis',(0.,-1.,0.));
#23752=DIRECTION('ref_axis',(0.,0.,1.));
#23753=DIRECTION('',(0.,-1.,0.));
#23754=DIRECTION('',(0.,1.,0.));
#23755=DIRECTION('center_axis',(-0.816496580927726,-0.408248290463866,-0.40824829046386));
#23756=DIRECTION('ref_axis',(-0.577350269189626,0.577350269189629,0.577350269189623));
#23757=DIRECTION('center_axis',(-1.,0.,0.));
#23758=DIRECTION('ref_axis',(0.,0.707106781186551,0.707106781186544));
#23759=DIRECTION('center_axis',(0.,0.,1.));
#23760=DIRECTION('ref_axis',(-0.707106781186544,0.707106781186551,0.));
#23761=DIRECTION('center_axis',(0.,1.,0.));
#23762=DIRECTION('ref_axis',(-0.707106781186545,0.,-0.70710678118655));
#23763=DIRECTION('center_axis',(0.,-1.,0.));
#23764=DIRECTION('ref_axis',(-1.,0.,0.));
#23765=DIRECTION('',(0.,-1.,0.));
#23766=DIRECTION('',(0.,1.,0.));
#23767=DIRECTION('center_axis',(-0.408248290463864,-0.816496580927727,-0.408248290463861));
#23768=DIRECTION('ref_axis',(-0.57735026918963,0.577350269189624,-0.577350269189624));
#23769=DIRECTION('center_axis',(0.,0.,-1.));
#23770=DIRECTION('ref_axis',(-0.707106781186544,0.707106781186551,0.));
#23771=DIRECTION('center_axis',(-1.,0.,0.));
#23772=DIRECTION('ref_axis',(0.,0.707106781186547,-0.707106781186547));
#23773=DIRECTION('center_axis',(0.,1.,0.));
#23774=DIRECTION('ref_axis',(-0.70710678118655,0.,0.707106781186545));
#23775=DIRECTION('center_axis',(0.,-1.,0.));
#23776=DIRECTION('ref_axis',(0.,0.,1.));
#23777=DIRECTION('',(0.,-1.,0.));
#23778=DIRECTION('',(0.,1.,0.));
#23779=DIRECTION('center_axis',(-0.408248290463864,-0.816496580927727,0.408248290463861));
#23780=DIRECTION('ref_axis',(-0.57735026918963,0.577350269189624,0.577350269189624));
#23781=DIRECTION('center_axis',(-1.,0.,0.));
#23782=DIRECTION('ref_axis',(0.,0.707106781186551,0.707106781186544));
#23783=DIRECTION('center_axis',(0.,0.,1.));
#23784=DIRECTION('ref_axis',(-0.707106781186544,0.707106781186551,0.));
#23785=DIRECTION('center_axis',(0.,1.,0.));
#23786=DIRECTION('ref_axis',(-0.923879532511286,0.,0.382683432365091));
#23787=DIRECTION('center_axis',(0.,-1.,0.));
#23788=DIRECTION('ref_axis',(-0.707106781186547,0.,0.707106781186547));
#23789=DIRECTION('',(0.,-1.,0.));
#23790=DIRECTION('',(0.,1.,0.));
#23791=DIRECTION('center_axis',(0.,0.,1.));
#23792=DIRECTION('ref_axis',(1.,0.,0.));
#23793=DIRECTION('center_axis',(-0.707106781186548,0.,-0.707106781186547));
#23794=DIRECTION('ref_axis',(-0.499999999999997,0.707106781186552,0.499999999999998));
#23795=DIRECTION('center_axis',(0.,0.,1.));
#23796=DIRECTION('ref_axis',(-0.707106781186545,0.70710678118655,0.));
#23797=DIRECTION('center_axis',(0.,1.,0.));
#23798=DIRECTION('ref_axis',(0.923879532511287,0.,0.382683432365088));
#23799=DIRECTION('',(0.,1.,0.));
#23800=DIRECTION('center_axis',(0.,-1.,0.));
#23801=DIRECTION('ref_axis',(1.,0.,0.));
#23802=DIRECTION('',(0.,-1.,0.));
#23803=DIRECTION('center_axis',(0.182143211721524,-0.879465224064608,0.43973261203231));
#23804=DIRECTION('ref_axis',(0.33655677059078,0.475963149477969,0.812519920068744));
#23805=DIRECTION('center_axis',(1.,0.,0.));
#23806=DIRECTION('ref_axis',(0.,0.707106781186551,0.707106781186544));
#23807=DIRECTION('center_axis',(0.,0.,1.));
#23808=DIRECTION('ref_axis',(1.,0.,0.));
#23809=DIRECTION('center_axis',(0.,0.,1.));
#23810=DIRECTION('ref_axis',(0.707106781186545,0.70710678118655,0.));
#23811=DIRECTION('center_axis',(0.,0.,1.));
#23812=DIRECTION('ref_axis',(-0.707106781186545,0.70710678118655,0.));
#23813=DIRECTION('center_axis',(0.,0.,-1.));
#23814=DIRECTION('ref_axis',(-1.,0.,0.));
#23815=DIRECTION('',(0.,0.,1.));
#23816=DIRECTION('center_axis',(0.707106781186548,0.,0.707106781186547));
#23817=DIRECTION('ref_axis',(-0.499999999999998,0.707106781186551,0.499999999999998));
#23818=DIRECTION('',(0.707106781186548,0.,0.707106781186547));
#23819=DIRECTION('center_axis',(0.382683432365088,0.,0.923879532511288));
#23820=DIRECTION('ref_axis',(0.923879532511288,0.,-0.382683432365088));
#23821=DIRECTION('center_axis',(-0.707106781186547,0.,0.707106781186548));
#23822=DIRECTION('ref_axis',(0.707106781186548,0.,0.707106781186547));
#23823=DIRECTION('',(0.,1.,0.));
#23824=DIRECTION('center_axis',(-1.,0.,0.));
#23825=DIRECTION('ref_axis',(0.,0.,1.));
#23826=DIRECTION('',(0.,0.,1.));
#23827=DIRECTION('center_axis',(0.,0.,1.));
#23828=DIRECTION('ref_axis',(-0.707106781186545,0.70710678118655,0.));
#23829=DIRECTION('center_axis',(1.,0.,0.));
#23830=DIRECTION('ref_axis',(0.,0.707106781186553,0.707106781186542));
#23831=DIRECTION('',(1.,0.,0.));
#23832=DIRECTION('center_axis',(0.707106781186548,0.,0.707106781186548));
#23833=DIRECTION('ref_axis',(0.707106781186548,0.,-0.707106781186548));
#23834=DIRECTION('center_axis',(0.,0.,1.));
#23835=DIRECTION('ref_axis',(1.,0.,0.));
#23836=DIRECTION('',(0.,1.,0.));
#23837=DIRECTION('center_axis',(-1.,0.,0.));
#23838=DIRECTION('ref_axis',(0.,0.,1.));
#23839=DIRECTION('',(0.,1.,0.));
#23840=DIRECTION('',(0.,0.,1.));
#23841=DIRECTION('center_axis',(0.,0.,-1.));
#23842=DIRECTION('ref_axis',(-1.,0.,0.));
#23843=DIRECTION('',(-1.,0.,0.));
#23844=DIRECTION('center_axis',(-1.,0.,0.));
#23845=DIRECTION('ref_axis',(0.,0.707106781186547,-0.707106781186547));
#23846=DIRECTION('center_axis',(-0.707106781186548,0.,0.707106781186548));
#23847=DIRECTION('ref_axis',(0.707106781186548,0.,0.707106781186548));
#23848=DIRECTION('center_axis',(-1.,0.,0.));
#23849=DIRECTION('ref_axis',(0.,0.,1.));
#23850=DIRECTION('',(0.,0.,1.));
#23851=DIRECTION('center_axis',(0.,0.,1.));
#23852=DIRECTION('ref_axis',(-0.707106781186545,0.70710678118655,0.));
#23853=DIRECTION('center_axis',(0.,0.,1.));
#23854=DIRECTION('ref_axis',(1.,0.,0.));
#23855=DIRECTION('',(1.,0.,0.));
#23856=DIRECTION('center_axis',(1.,0.,0.));
#23857=DIRECTION('ref_axis',(0.,0.707106781186547,0.707106781186547));
#23858=DIRECTION('center_axis',(0.707106781186548,0.,0.707106781186547));
#23859=DIRECTION('ref_axis',(0.707106781186547,0.,-0.707106781186548));
#23860=DIRECTION('center_axis',(0.,0.,1.));
#23861=DIRECTION('ref_axis',(-0.707106781186545,0.70710678118655,0.));
#23862=DIRECTION('center_axis',(0.,0.,-1.));
#23863=DIRECTION('ref_axis',(0.707106781186545,0.70710678118655,0.));
#23864=DIRECTION('',(0.,0.,-1.));
#23865=DIRECTION('center_axis',(0.,0.,1.));
#23866=DIRECTION('ref_axis',(1.,0.,0.));
#23867=DIRECTION('center_axis',(0.,-1.,0.));
#23868=DIRECTION('ref_axis',(0.,0.,-1.));
#23869=DIRECTION('center_axis',(0.,-1.,0.));
#23870=DIRECTION('ref_axis',(6.46422633350345E-16,0.,-1.));
#23871=DIRECTION('center_axis',(-1.,0.,0.));
#23872=DIRECTION('ref_axis',(0.,0.,1.));
#23873=DIRECTION('',(0.,1.,0.));
#23874=DIRECTION('center_axis',(0.,1.,0.));
#23875=DIRECTION('ref_axis',(1.,0.,5.85190293392977E-16));
#23876=DIRECTION('',(0.,1.,0.));
#23877=DIRECTION('center_axis',(1.,0.,0.));
#23878=DIRECTION('ref_axis',(0.,0.,-1.));
#23879=DIRECTION('center_axis',(1.,0.,0.));
#23880=DIRECTION('ref_axis',(0.,0.707106781186553,0.707106781186542));
#23881=DIRECTION('center_axis',(0.,-1.,0.));
#23882=DIRECTION('ref_axis',(0.,0.,-1.));
#23883=DIRECTION('center_axis',(0.,-1.,0.));
#23884=DIRECTION('ref_axis',(-0.707106781186547,0.,-0.707106781186548));
#23885=DIRECTION('center_axis',(0.,0.,-1.));
#23886=DIRECTION('ref_axis',(0.707106781186545,0.70710678118655,0.));
#23887=DIRECTION('',(0.,0.,-1.));
#23888=DIRECTION('center_axis',(0.,1.,0.));
#23889=DIRECTION('ref_axis',(-0.707106781186547,0.,-0.707106781186547));
#23890=DIRECTION('center_axis',(-1.,0.,0.));
#23891=DIRECTION('ref_axis',(0.,0.,1.));
#23892=DIRECTION('center_axis',(0.,-1.,0.));
#23893=DIRECTION('ref_axis',(0.,0.,-1.));
#23894=DIRECTION('center_axis',(-1.,0.,0.));
#23895=DIRECTION('ref_axis',(0.,0.,1.));
#23896=DIRECTION('center_axis',(0.,0.,1.));
#23897=DIRECTION('ref_axis',(-0.707106781186544,0.707106781186551,0.));
#23898=DIRECTION('center_axis',(0.,0.,1.));
#23899=DIRECTION('ref_axis',(0.,1.,0.));
#23900=DIRECTION('center_axis',(0.,0.,-1.));
#23901=DIRECTION('ref_axis',(-1.,0.,0.));
#23902=DIRECTION('center_axis',(0.,-1.,0.));
#23903=DIRECTION('ref_axis',(1.65389215948551E-15,0.,1.));
#23904=DIRECTION('center_axis',(0.,0.,1.));
#23905=DIRECTION('ref_axis',(1.,0.,0.));
#23906=DIRECTION('center_axis',(0.,-1.,0.));
#23907=DIRECTION('ref_axis',(1.49370186820111E-15,0.,1.));
#23908=DIRECTION('center_axis',(0.,0.,-1.));
#23909=DIRECTION('ref_axis',(0.707106781186544,0.707106781186551,0.));
#23910=DIRECTION('center_axis',(0.,0.,1.));
#23911=DIRECTION('ref_axis',(1.,0.,0.));
#23912=DIRECTION('',(0.,0.,-1.));
#23913=DIRECTION('center_axis',(0.,-1.,0.));
#23914=DIRECTION('ref_axis',(0.,0.,-1.));
#23915=DIRECTION('center_axis',(0.,1.,0.));
#23916=DIRECTION('ref_axis',(-1.,0.,1.55493420815848E-15));
#23917=DIRECTION('',(0.,1.,0.));
#23918=DIRECTION('center_axis',(0.,1.,0.));
#23919=DIRECTION('ref_axis',(0.,0.,1.));
#23920=DIRECTION('center_axis',(-1.,0.,0.));
#23921=DIRECTION('ref_axis',(0.,0.,-1.));
#23922=DIRECTION('center_axis',(0.,1.,0.));
#23923=DIRECTION('ref_axis',(0.,0.,1.));
#23924=DIRECTION('center_axis',(0.,-1.,0.));
#23925=DIRECTION('ref_axis',(1.,0.,0.));
#23926=DIRECTION('center_axis',(-1.,0.,0.));
#23927=DIRECTION('ref_axis',(0.,0.,-1.));
#23928=DIRECTION('center_axis',(0.,-1.,0.));
#23929=DIRECTION('ref_axis',(1.,0.,0.));
#23930=DIRECTION('center_axis',(0.,1.,0.));
#23931=DIRECTION('ref_axis',(1.,0.,0.));
#23932=DIRECTION('center_axis',(0.,1.,1.15415719212674E-15));
#23933=DIRECTION('ref_axis',(1.,0.,0.));
#23934=DIRECTION('center_axis',(0.,1.,1.15415719212674E-15));
#23935=DIRECTION('ref_axis',(1.,0.,0.));
#23936=DIRECTION('',(-0.707106781186547,0.707106781186548,8.65956056235493E-17));
#23937=DIRECTION('center_axis',(0.,-1.,0.));
#23938=DIRECTION('ref_axis',(0.,0.,-1.));
#23939=DIRECTION('center_axis',(-1.,0.,0.));
#23940=DIRECTION('ref_axis',(0.,0.,1.));
#23941=DIRECTION('center_axis',(-1.,0.,0.));
#23942=DIRECTION('ref_axis',(0.,0.,1.));
#23943=DIRECTION('center_axis',(0.707106781186547,0.,0.707106781186548));
#23944=DIRECTION('ref_axis',(0.707106781186548,0.,-0.707106781186547));
#59065=CARTESIAN_POINT('',(0.,0.,0.));
#59066=CARTESIAN_POINT('Origin',(-29.376,24.6394718625761,38.352));
#59067=CARTESIAN_POINT('',(-33.2237359312881,25.0637359312881,38.352));
#59068=CARTESIAN_POINT('',(-29.376,25.0637359312881,42.1997359312881));
#59069=CARTESIAN_POINT('Origin',(-29.376,25.0637359312881,38.352));
#59070=CARTESIAN_POINT('',(-29.376,24.6394718625761,42.024));
#59071=CARTESIAN_POINT('Origin',(-29.376,24.6394718625761,42.624));
#59072=CARTESIAN_POINT('',(-33.048,24.6394718625761,38.352));
#59073=CARTESIAN_POINT('Origin',(-29.376,24.6394718625761,38.352));
#59074=CARTESIAN_POINT('Origin',(-29.376,24.6394718625761,38.352));
#59075=CARTESIAN_POINT('Origin',(-29.376,25.0637359312881,38.352));
#59076=CARTESIAN_POINT('Origin',(-29.376,22.44,38.352));
#59077=CARTESIAN_POINT('',(-29.376,23.04,34.68));
#59078=CARTESIAN_POINT('',(-33.048,23.04,38.352));
#59079=CARTESIAN_POINT('Origin',(-29.376,23.04,38.352));
#59080=CARTESIAN_POINT('Origin',(-29.376,23.04,38.352));
#59081=CARTESIAN_POINT('',(-33.048,22.44,38.352));
#59082=CARTESIAN_POINT('Origin',(-29.376,25.296,38.352));
#59083=CARTESIAN_POINT('',(-33.6882640687119,25.5282640687119,38.352));
#59084=CARTESIAN_POINT('',(-33.456,25.296,38.352));
#59085=CARTESIAN_POINT('',(-29.376,25.5282640687119,34.0397359312881));
#59086=CARTESIAN_POINT('Origin',(-29.376,25.5282640687119,38.352));
#59087=CARTESIAN_POINT('Origin',(-29.376,25.5282640687119,38.352));
#59088=CARTESIAN_POINT('Origin',(-17.352,22.44,6.82615721505037));
#59089=CARTESIAN_POINT('',(-17.952,23.04,6.82615721505037));
#59090=CARTESIAN_POINT('',(-17.5132903225806,23.04,7.40407194218736));
#59091=CARTESIAN_POINT('Origin',(-17.352,23.04,6.82615721505037));
#59092=CARTESIAN_POINT('',(-17.5132903225806,25.104,7.40407194218736));
#59093=CARTESIAN_POINT('',(-17.5132903225806,22.44,7.40407194218736));
#59094=CARTESIAN_POINT('',(-17.952,25.104,6.82615721505037));
#59095=CARTESIAN_POINT('Origin',(-17.352,25.104,6.82615721505037));
#59096=CARTESIAN_POINT('',(-17.952,22.44,6.82615721505037));
#59097=CARTESIAN_POINT('Origin',(-17.352,25.104,6.82615721505037));
#59098=CARTESIAN_POINT('',(-17.352,25.704,6.82615721505037));
#59099=CARTESIAN_POINT('Origin',(-17.352,25.104,6.82615721505037));
#59100=CARTESIAN_POINT('Origin',(-17.352,25.104,6.82615721505037));
#59101=CARTESIAN_POINT('Origin',(-17.352,23.04,6.82615721505037));
#59102=CARTESIAN_POINT('',(-17.352,22.44,6.82615721505037));
#59103=CARTESIAN_POINT('Origin',(-17.352,23.04,6.82615721505037));
#59104=CARTESIAN_POINT('Origin',(-17.352,23.04,6.82615721505037));
#59105=CARTESIAN_POINT('Origin',(-17.352,25.104,5.1));
#59106=CARTESIAN_POINT('',(-17.352,25.704,-32.9381572150504));
#59107=CARTESIAN_POINT('',(-17.352,25.704,5.1));
#59108=CARTESIAN_POINT('',(-17.952,25.104,-32.9381572150504));
#59109=CARTESIAN_POINT('Origin',(-17.352,25.104,-32.9381572150504));
#59110=CARTESIAN_POINT('',(-17.952,25.104,5.1));
#59111=CARTESIAN_POINT('Origin',(-17.952,25.104,8.976));
#59112=CARTESIAN_POINT('',(-19.5239280578126,25.104,9.41470967741935));
#59113=CARTESIAN_POINT('Origin',(-17.952,25.104,8.976));
#59114=CARTESIAN_POINT('',(-20.1018427849496,25.704,9.576));
#59115=CARTESIAN_POINT('Origin',(-20.1018427849496,25.104,9.576));
#59116=CARTESIAN_POINT('Origin',(-17.952,25.704,8.976));
#59117=CARTESIAN_POINT('Origin',(-17.952,22.44,8.976));
#59118=CARTESIAN_POINT('',(-19.5239280578126,23.04,9.41470967741935));
#59119=CARTESIAN_POINT('Origin',(-17.952,23.04,8.976));
#59120=CARTESIAN_POINT('',(-19.5239280578126,22.44,9.41470967741935));
#59121=CARTESIAN_POINT('Origin',(-17.352,22.44,-32.9381572150504));
#59122=CARTESIAN_POINT('',(-17.5132903225806,25.104,-33.5160719421874));
#59123=CARTESIAN_POINT('Origin',(-17.352,25.104,-32.9381572150504));
#59124=CARTESIAN_POINT('',(-17.5132903225806,23.04,-33.5160719421874));
#59125=CARTESIAN_POINT('',(-17.5132903225806,22.44,-33.5160719421874));
#59126=CARTESIAN_POINT('',(-17.952,23.04,-32.9381572150504));
#59127=CARTESIAN_POINT('Origin',(-17.352,23.04,-32.9381572150504));
#59128=CARTESIAN_POINT('',(-17.952,22.44,-32.9381572150504));
#59129=CARTESIAN_POINT('Origin',(-17.352,23.04,-32.9381572150504));
#59130=CARTESIAN_POINT('',(-17.352,22.44,-32.9381572150504));
#59131=CARTESIAN_POINT('Origin',(-17.352,23.04,-32.9381572150504));
#59132=CARTESIAN_POINT('Origin',(-17.352,23.04,-32.9381572150504));
#59133=CARTESIAN_POINT('Origin',(-17.352,25.104,-32.9381572150504));
#59134=CARTESIAN_POINT('Origin',(-17.352,25.104,-32.9381572150504));
#59135=CARTESIAN_POINT('Origin',(-17.952,25.104,-35.088));
#59136=CARTESIAN_POINT('',(-20.1018427849496,25.704,-35.688));
#59137=CARTESIAN_POINT('Origin',(-17.952,25.704,-35.088));
#59138=CARTESIAN_POINT('',(-19.5239280578126,25.104,-35.5267096774194));
#59139=CARTESIAN_POINT('Origin',(-20.1018427849496,25.104,-35.688));
#59140=CARTESIAN_POINT('Origin',(-17.952,25.104,-35.088));
#59141=CARTESIAN_POINT('Origin',(-17.952,22.44,8.976));
#59142=CARTESIAN_POINT('',(-17.952,23.04,5.1));
#59143=CARTESIAN_POINT('Origin',(-20.1018427849496,22.44,-35.688));
#59144=CARTESIAN_POINT('',(-20.1018427849496,23.04,-35.088));
#59145=CARTESIAN_POINT('',(-19.5239280578126,23.04,-35.5267096774194));
#59146=CARTESIAN_POINT('Origin',(-20.1018427849496,23.04,-35.688));
#59147=CARTESIAN_POINT('',(-19.5239280578126,22.44,-35.5267096774194));
#59148=CARTESIAN_POINT('',(-20.1018427849496,25.104,-35.088));
#59149=CARTESIAN_POINT('Origin',(-20.1018427849496,25.104,-35.688));
#59150=CARTESIAN_POINT('',(-20.1018427849496,22.44,-35.088));
#59151=CARTESIAN_POINT('Origin',(-20.1018427849496,25.104,-35.688));
#59152=CARTESIAN_POINT('Origin',(-20.1018427849496,25.104,-35.688));
#59153=CARTESIAN_POINT('Origin',(-20.1018427849496,23.04,-35.688));
#59154=CARTESIAN_POINT('',(-20.1018427849496,22.44,-35.688));
#59155=CARTESIAN_POINT('Origin',(-20.1018427849496,23.04,-35.688));
#59156=CARTESIAN_POINT('Origin',(-20.1018427849496,23.04,-35.688));
#59157=CARTESIAN_POINT('Origin',(-8.976,25.104,-35.688));
#59158=CARTESIAN_POINT('',(-26.4101572150504,25.704,-35.688));
#59159=CARTESIAN_POINT('',(-8.976,25.704,-35.688));
#59160=CARTESIAN_POINT('',(-26.4101572150504,25.104,-35.088));
#59161=CARTESIAN_POINT('Origin',(-26.4101572150504,25.104,-35.688));
#59162=CARTESIAN_POINT('',(-8.976,25.104,-35.088));
#59163=CARTESIAN_POINT('Origin',(-17.952,22.44,-35.088));
#59164=CARTESIAN_POINT('Origin',(-17.952,23.04,-35.088));
#59165=CARTESIAN_POINT('Origin',(-26.4101572150504,22.44,-35.688));
#59166=CARTESIAN_POINT('',(-26.9880719421874,25.104,-35.5267096774194));
#59167=CARTESIAN_POINT('Origin',(-26.4101572150504,25.104,-35.688));
#59168=CARTESIAN_POINT('',(-26.9880719421874,23.04,-35.5267096774194));
#59169=CARTESIAN_POINT('',(-26.9880719421874,22.44,-35.5267096774194));
#59170=CARTESIAN_POINT('',(-26.4101572150504,23.04,-35.088));
#59171=CARTESIAN_POINT('Origin',(-26.4101572150504,23.04,-35.688));
#59172=CARTESIAN_POINT('',(-26.4101572150504,22.44,-35.088));
#59173=CARTESIAN_POINT('Origin',(-26.4101572150504,23.04,-35.688));
#59174=CARTESIAN_POINT('',(-26.4101572150504,22.44,-35.688));
#59175=CARTESIAN_POINT('Origin',(-26.4101572150504,23.04,-35.688));
#59176=CARTESIAN_POINT('Origin',(-26.4101572150504,23.04,-35.688));
#59177=CARTESIAN_POINT('Origin',(-26.4101572150504,25.104,-35.688));
#59178=CARTESIAN_POINT('Origin',(-26.4101572150504,25.104,-35.688));
#59179=CARTESIAN_POINT('Origin',(-28.56,25.104,-35.088));
#59180=CARTESIAN_POINT('',(-29.16,25.704,-32.9381572150504));
#59181=CARTESIAN_POINT('Origin',(-28.56,25.704,-35.088));
#59182=CARTESIAN_POINT('',(-28.9987096774194,25.104,-33.5160719421874));
#59183=CARTESIAN_POINT('Origin',(-29.16,25.104,-32.9381572150504));
#59184=CARTESIAN_POINT('Origin',(-28.56,25.104,-35.088));
#59185=CARTESIAN_POINT('Origin',(-17.952,22.44,-35.088));
#59186=CARTESIAN_POINT('',(-8.976,23.04,-35.088));
#59187=CARTESIAN_POINT('Origin',(26.4101572150504,22.44,9.576));
#59188=CARTESIAN_POINT('',(26.4101572150504,25.104,8.976));
#59189=CARTESIAN_POINT('',(26.9880719421874,25.104,9.41470967741935));
#59190=CARTESIAN_POINT('Origin',(26.4101572150504,25.104,9.576));
#59191=CARTESIAN_POINT('',(26.9880719421874,23.04,9.41470967741935));
#59192=CARTESIAN_POINT('',(26.9880719421874,22.44,9.41470967741935));
#59193=CARTESIAN_POINT('',(26.4101572150504,23.04,8.976));
#59194=CARTESIAN_POINT('Origin',(26.4101572150504,23.04,9.576));
#59195=CARTESIAN_POINT('',(26.4101572150504,22.44,8.976));
#59196=CARTESIAN_POINT('Origin',(26.4101572150504,23.04,9.576));
#59197=CARTESIAN_POINT('',(26.4101572150504,22.44,9.576));
#59198=CARTESIAN_POINT('Origin',(26.4101572150504,23.04,9.576));
#59199=CARTESIAN_POINT('Origin',(26.4101572150504,23.04,9.576));
#59200=CARTESIAN_POINT('Origin',(26.4101572150504,25.104,9.576));
#59201=CARTESIAN_POINT('',(26.4101572150504,25.704,9.576));
#59202=CARTESIAN_POINT('Origin',(26.4101572150504,25.104,9.576));
#59203=CARTESIAN_POINT('Origin',(26.4101572150504,25.104,9.576));
#59204=CARTESIAN_POINT('Origin',(28.56,25.104,8.976));
#59205=CARTESIAN_POINT('',(29.16,25.704,6.82615721505037));
#59206=CARTESIAN_POINT('Origin',(28.56,25.704,8.976));
#59207=CARTESIAN_POINT('',(28.9987096774193,25.104,7.40407194218736));
#59208=CARTESIAN_POINT('Origin',(29.16,25.104,6.82615721505037));
#59209=CARTESIAN_POINT('Origin',(28.56,25.104,8.976));
#59210=CARTESIAN_POINT('Origin',(8.976,25.104,9.576));
#59211=CARTESIAN_POINT('',(20.1018427849496,25.104,8.976));
#59212=CARTESIAN_POINT('',(8.976,25.104,8.976));
#59213=CARTESIAN_POINT('',(20.1018427849496,25.704,9.576));
#59214=CARTESIAN_POINT('Origin',(20.1018427849496,25.104,9.576));
#59215=CARTESIAN_POINT('',(8.976,25.704,9.576));
#59216=CARTESIAN_POINT('Origin',(17.952,22.44,8.976));
#59217=CARTESIAN_POINT('',(20.1018427849496,23.04,8.976));
#59218=CARTESIAN_POINT('',(8.976,23.04,8.976));
#59219=CARTESIAN_POINT('',(20.1018427849496,22.44,8.976));
#59220=CARTESIAN_POINT('Origin',(29.16,22.44,6.82615721505037));
#59221=CARTESIAN_POINT('',(28.56,23.04,6.82615721505037));
#59222=CARTESIAN_POINT('',(28.9987096774193,23.04,7.40407194218736));
#59223=CARTESIAN_POINT('Origin',(29.16,23.04,6.82615721505037));
#59224=CARTESIAN_POINT('',(28.9987096774193,22.44,7.40407194218736));
#59225=CARTESIAN_POINT('',(28.56,25.104,6.82615721505037));
#59226=CARTESIAN_POINT('Origin',(29.16,25.104,6.82615721505037));
#59227=CARTESIAN_POINT('',(28.56,22.44,6.82615721505037));
#59228=CARTESIAN_POINT('Origin',(29.16,25.104,6.82615721505037));
#59229=CARTESIAN_POINT('Origin',(29.16,25.104,6.82615721505037));
#59230=CARTESIAN_POINT('Origin',(29.16,23.04,6.82615721505037));
#59231=CARTESIAN_POINT('',(29.16,22.44,6.82615721505037));
#59232=CARTESIAN_POINT('Origin',(29.16,23.04,6.82615721505037));
#59233=CARTESIAN_POINT('Origin',(29.16,23.04,6.82615721505037));
#59234=CARTESIAN_POINT('Origin',(29.16,25.104,5.1));
#59235=CARTESIAN_POINT('',(29.16,25.704,-32.9381572150504));
#59236=CARTESIAN_POINT('',(29.16,25.704,5.1));
#59237=CARTESIAN_POINT('',(28.56,25.104,-32.9381572150504));
#59238=CARTESIAN_POINT('Origin',(29.16,25.104,-32.9381572150504));
#59239=CARTESIAN_POINT('',(28.56,25.104,5.1));
#59240=CARTESIAN_POINT('Origin',(28.56,22.44,8.976));
#59241=CARTESIAN_POINT('Origin',(28.56,23.04,8.976));
#59242=CARTESIAN_POINT('Origin',(-28.152,23.04,28.56));
#59243=CARTESIAN_POINT('',(-28.152,22.44,25.46));
#59244=CARTESIAN_POINT('Origin',(-28.152,22.44,28.56));
#59245=CARTESIAN_POINT('',(-28.152,23.04,26.06));
#59246=CARTESIAN_POINT('Origin',(-28.152,23.04,25.46));
#59247=CARTESIAN_POINT('',(-30.652,23.04,28.56));
#59248=CARTESIAN_POINT('Origin',(-28.152,23.04,28.56));
#59249=CARTESIAN_POINT('Origin',(-28.152,23.04,28.56));
#59250=CARTESIAN_POINT('Origin',(0.,22.44,1.224));
#59251=CARTESIAN_POINT('',(-14.472,22.44,12.8074718625761));
#59252=CARTESIAN_POINT('',(-8.1888,22.44,6.52427186257614));
#59253=CARTESIAN_POINT('',(-7.87026406871193,22.44,6.20573593128807));
#59254=CARTESIAN_POINT('',(-14.472,22.44,32.448));
#59255=CARTESIAN_POINT('',(-14.472,22.44,17.136));
#59256=CARTESIAN_POINT('',(-17.328,22.44,32.448));
#59257=CARTESIAN_POINT('',(-8.364,22.44,32.448));
#59258=CARTESIAN_POINT('',(-17.328,22.44,39.768));
#59259=CARTESIAN_POINT('',(-17.328,22.44,20.196));
#59260=CARTESIAN_POINT('',(-14.472,22.44,39.768));
#59261=CARTESIAN_POINT('',(-6.936,22.44,39.768));
#59262=CARTESIAN_POINT('',(-14.472,22.44,47.952));
#59263=CARTESIAN_POINT('',(-14.472,22.44,24.888));
#59264=CARTESIAN_POINT('',(-32.3914718625761,22.44,47.952));
#59265=CARTESIAN_POINT('',(-16.32,22.44,47.952));
#59266=CARTESIAN_POINT('',(-35.712,22.44,44.6314718625761));
#59267=CARTESIAN_POINT('',(-37.7237359312881,22.44,42.619735931288));
#59268=CARTESIAN_POINT('',(-35.712,22.44,-42.2038804065906));
#59269=CARTESIAN_POINT('',(-35.712,22.44,-20.604));
#59270=CARTESIAN_POINT('',(-32.7785603614138,22.44,-45.504));
#59271=CARTESIAN_POINT('',(-37.0566026846519,22.44,-40.6912023863572));
#59272=CARTESIAN_POINT('',(32.7785603614138,22.44,-45.504));
#59273=CARTESIAN_POINT('',(16.524,22.44,-45.504));
#59274=CARTESIAN_POINT('',(35.712,22.44,-42.2038804065906));
#59275=CARTESIAN_POINT('',(38.6886026846519,22.44,-38.8552023863572));
#59276=CARTESIAN_POINT('',(35.712,22.44,44.6314718625761));
#59277=CARTESIAN_POINT('',(35.712,22.44,23.052));
#59278=CARTESIAN_POINT('',(32.3914718625761,22.44,47.952));
#59279=CARTESIAN_POINT('',(35.8877359312881,22.44,44.455735931288));
#59280=CARTESIAN_POINT('',(14.472,22.44,47.952));
#59281=CARTESIAN_POINT('',(6.936,22.44,47.952));
#59282=CARTESIAN_POINT('',(14.472,22.44,39.768));
#59283=CARTESIAN_POINT('',(14.472,22.44,20.196));
#59284=CARTESIAN_POINT('',(17.328,22.44,39.768));
#59285=CARTESIAN_POINT('',(8.364,22.44,39.768));
#59286=CARTESIAN_POINT('',(17.328,22.44,32.448));
#59287=CARTESIAN_POINT('',(17.328,22.44,17.136));
#59288=CARTESIAN_POINT('',(14.472,22.44,32.448));
#59289=CARTESIAN_POINT('',(6.936,22.44,32.448));
#59290=CARTESIAN_POINT('',(14.472,22.44,12.8074718625761));
#59291=CARTESIAN_POINT('',(14.472,22.44,7.14));
#59292=CARTESIAN_POINT('',(8.1888,22.44,6.52427186257615));
#59293=CARTESIAN_POINT('',(4.72866406871193,22.44,3.06413593128807));
#59294=CARTESIAN_POINT('',(8.1888,22.44,-21.7872));
#59295=CARTESIAN_POINT('',(8.1888,22.44,-10.2816));
#59296=CARTESIAN_POINT('',(-8.1888,22.44,-21.7872));
#59297=CARTESIAN_POINT('Origin',(0.,22.44,-21.7872));
#59298=CARTESIAN_POINT('',(-8.1888,22.44,3.9984));
#59299=CARTESIAN_POINT('',(29.376,22.44,34.08));
#59300=CARTESIAN_POINT('Origin',(29.376,22.44,38.352));
#59301=CARTESIAN_POINT('',(3.456,22.44,-37.944));
#59302=CARTESIAN_POINT('',(3.456,22.44,-35.496));
#59303=CARTESIAN_POINT('',(3.456,22.44,-17.136));
#59304=CARTESIAN_POINT('',(-3.456,22.44,-37.944));
#59305=CARTESIAN_POINT('Origin',(0.,22.44,-37.944));
#59306=CARTESIAN_POINT('',(-3.456,22.44,-35.496));
#59307=CARTESIAN_POINT('',(-3.456,22.44,-18.36));
#59308=CARTESIAN_POINT('Origin',(0.,22.44,-35.496));
#59309=CARTESIAN_POINT('',(29.16,22.44,-32.9381572150504));
#59310=CARTESIAN_POINT('',(29.16,22.44,5.1));
#59311=CARTESIAN_POINT('',(26.4101572150504,22.44,-35.688));
#59312=CARTESIAN_POINT('Origin',(28.56,22.44,-35.088));
#59313=CARTESIAN_POINT('',(20.1018427849496,22.44,-35.688));
#59314=CARTESIAN_POINT('',(14.28,22.44,-35.688));
#59315=CARTESIAN_POINT('',(17.352,22.44,-32.9381572150504));
#59316=CARTESIAN_POINT('Origin',(17.952,22.44,-35.088));
#59317=CARTESIAN_POINT('',(17.352,22.44,6.82615721505036));
#59318=CARTESIAN_POINT('',(17.352,22.44,-16.932));
#59319=CARTESIAN_POINT('',(20.1018427849496,22.44,9.576));
#59320=CARTESIAN_POINT('Origin',(17.952,22.44,8.976));
#59321=CARTESIAN_POINT('',(8.976,22.44,9.576));
#59322=CARTESIAN_POINT('Origin',(28.56,22.44,8.976));
#59323=CARTESIAN_POINT('',(28.152,22.44,25.46));
#59324=CARTESIAN_POINT('Origin',(28.152,22.44,28.56));
#59325=CARTESIAN_POINT('',(-26.4101572150504,22.44,9.576));
#59326=CARTESIAN_POINT('',(-29.16,22.44,6.82615721505037));
#59327=CARTESIAN_POINT('Origin',(-28.56,22.44,8.976));
#59328=CARTESIAN_POINT('',(-20.1018427849496,22.44,9.576));
#59329=CARTESIAN_POINT('',(-14.28,22.44,9.576));
#59330=CARTESIAN_POINT('Origin',(-17.952,22.44,8.976));
#59331=CARTESIAN_POINT('',(-17.352,22.44,5.1));
#59332=CARTESIAN_POINT('Origin',(-17.952,22.44,-35.088));
#59333=CARTESIAN_POINT('',(-8.976,22.44,-35.688));
#59334=CARTESIAN_POINT('',(-29.16,22.44,-32.9381572150504));
#59335=CARTESIAN_POINT('Origin',(-28.56,22.44,-35.088));
#59336=CARTESIAN_POINT('',(-29.16,22.44,-16.932));
#59337=CARTESIAN_POINT('',(-29.376,22.44,34.08));
#59338=CARTESIAN_POINT('Origin',(-29.376,22.44,38.352));
#59339=CARTESIAN_POINT('Origin',(-28.152,22.44,28.56));
#59340=CARTESIAN_POINT('',(-30.652,25.104,28.56));
#59341=CARTESIAN_POINT('',(-30.652,22.44,28.56));
#59342=CARTESIAN_POINT('',(-28.152,25.104,31.06));
#59343=CARTESIAN_POINT('Origin',(-28.152,25.104,28.56));
#59344=CARTESIAN_POINT('Origin',(-28.152,25.104,28.56));
#59345=CARTESIAN_POINT('Origin',(29.376,23.04,38.352));
#59346=CARTESIAN_POINT('',(29.376,23.04,34.68));
#59347=CARTESIAN_POINT('Origin',(29.376,23.04,34.08));
#59348=CARTESIAN_POINT('',(25.704,23.04,38.352));
#59349=CARTESIAN_POINT('Origin',(29.376,23.04,38.352));
#59350=CARTESIAN_POINT('Origin',(29.376,23.04,38.352));
#59351=CARTESIAN_POINT('Origin',(29.376,22.44,38.352));
#59352=CARTESIAN_POINT('',(25.704,24.6394718625761,38.352));
#59353=CARTESIAN_POINT('',(25.704,22.44,38.352));
#59354=CARTESIAN_POINT('',(29.376,24.6394718625761,42.024));
#59355=CARTESIAN_POINT('Origin',(29.376,24.6394718625761,38.352));
#59356=CARTESIAN_POINT('Origin',(29.376,24.6394718625761,38.352));
#59357=CARTESIAN_POINT('Origin',(-29.376,23.04,38.352));
#59358=CARTESIAN_POINT('Origin',(-29.376,23.04,34.08));
#59359=CARTESIAN_POINT('Origin',(3.456,23.04,-17.136));
#59360=CARTESIAN_POINT('',(2.856,23.04,-35.496));
#59361=CARTESIAN_POINT('Origin',(3.456,23.04,-35.496));
#59362=CARTESIAN_POINT('',(2.856,23.04,-37.944));
#59363=CARTESIAN_POINT('',(2.856,23.04,-17.136));
#59364=CARTESIAN_POINT('Origin',(3.456,23.04,-37.944));
#59365=CARTESIAN_POINT('Origin',(0.,23.04,-37.944));
#59366=CARTESIAN_POINT('',(-2.856,23.04,-37.944));
#59367=CARTESIAN_POINT('Origin',(-3.456,23.04,-37.944));
#59368=CARTESIAN_POINT('Origin',(0.,23.04,-37.944));
#59369=CARTESIAN_POINT('Origin',(-3.456,23.04,-18.36));
#59370=CARTESIAN_POINT('',(-2.856,23.04,-35.496));
#59371=CARTESIAN_POINT('Origin',(-3.456,23.04,-35.496));
#59372=CARTESIAN_POINT('',(-2.856,23.04,-18.36));
#59373=CARTESIAN_POINT('Origin',(0.,23.04,-35.496));
#59374=CARTESIAN_POINT('Origin',(0.,23.04,-35.496));
#59375=CARTESIAN_POINT('Origin',(0.,22.44,-37.944));
#59376=CARTESIAN_POINT('',(2.856,25.104,-37.944));
#59377=CARTESIAN_POINT('',(2.856,22.44,-37.944));
#59378=CARTESIAN_POINT('',(-2.856,25.104,-37.944));
#59379=CARTESIAN_POINT('Origin',(0.,25.104,-37.944));
#59380=CARTESIAN_POINT('',(-2.856,22.44,-37.944));
#59381=CARTESIAN_POINT('Origin',(2.856,22.44,-35.496));
#59382=CARTESIAN_POINT('',(2.856,25.104,-35.496));
#59383=CARTESIAN_POINT('',(2.856,22.44,-35.496));
#59384=CARTESIAN_POINT('',(2.856,25.104,-17.136));
#59385=CARTESIAN_POINT('Origin',(29.16,23.04,5.1));
#59386=CARTESIAN_POINT('',(28.56,23.04,-32.9381572150504));
#59387=CARTESIAN_POINT('',(28.56,23.04,5.1));
#59388=CARTESIAN_POINT('Origin',(29.16,23.04,-32.9381572150504));
#59389=CARTESIAN_POINT('Origin',(28.56,23.04,8.976));
#59390=CARTESIAN_POINT('Origin',(20.1018427849496,23.04,9.576));
#59391=CARTESIAN_POINT('Origin',(20.1018427849496,23.04,9.576));
#59392=CARTESIAN_POINT('',(19.5239280578126,23.04,9.41470967741935));
#59393=CARTESIAN_POINT('Origin',(20.1018427849496,23.04,9.576));
#59394=CARTESIAN_POINT('Origin',(20.1018427849496,23.04,9.576));
#59395=CARTESIAN_POINT('Origin',(8.976,23.04,9.576));
#59396=CARTESIAN_POINT('Origin',(29.16,23.04,-32.9381572150504));
#59397=CARTESIAN_POINT('',(28.9987096774193,23.04,-33.5160719421874));
#59398=CARTESIAN_POINT('Origin',(29.16,23.04,-32.9381572150504));
#59399=CARTESIAN_POINT('Origin',(29.16,23.04,-32.9381572150504));
#59400=CARTESIAN_POINT('Origin',(28.56,22.44,8.976));
#59401=CARTESIAN_POINT('',(28.56,22.44,-32.9381572150504));
#59402=CARTESIAN_POINT('Origin',(20.1018427849496,22.44,9.576));
#59403=CARTESIAN_POINT('',(19.5239280578126,25.104,9.41470967741935));
#59404=CARTESIAN_POINT('',(19.5239280578126,22.44,9.41470967741935));
#59405=CARTESIAN_POINT('Origin',(20.1018427849496,25.104,9.576));
#59406=CARTESIAN_POINT('Origin',(17.952,23.04,8.976));
#59407=CARTESIAN_POINT('',(17.5132903225806,23.04,7.40407194218736));
#59408=CARTESIAN_POINT('Origin',(17.352,23.04,6.82615721505037));
#59409=CARTESIAN_POINT('Origin',(17.952,23.04,8.976));
#59410=CARTESIAN_POINT('Origin',(-7.87026406871193,23.04,6.20573593128807));
#59411=CARTESIAN_POINT('',(-13.872,23.04,13.056));
#59412=CARTESIAN_POINT('Origin',(-14.472,23.04,12.8074718625761));
#59413=CARTESIAN_POINT('',(-7.76453593128807,23.04,6.94853593128807));
#59414=CARTESIAN_POINT('Origin',(-8.1888,23.04,6.52427186257614));
#59415=CARTESIAN_POINT('',(-7.446,23.04,6.63));
#59416=CARTESIAN_POINT('Origin',(-8.1888,23.04,6.52427186257615));
#59417=CARTESIAN_POINT('',(-7.5888,23.04,6.52427186257615));
#59418=CARTESIAN_POINT('Origin',(-8.1888,23.04,6.52427186257615));
#59419=CARTESIAN_POINT('Origin',(-8.1888,23.04,6.52427186257615));
#59420=CARTESIAN_POINT('Origin',(-8.1888,23.04,3.9984));
#59421=CARTESIAN_POINT('',(-7.5888,23.04,-21.7872));
#59422=CARTESIAN_POINT('Origin',(-8.1888,23.04,-21.7872));
#59423=CARTESIAN_POINT('',(-7.5888,23.04,3.9984));
#59424=CARTESIAN_POINT('Origin',(35.712,23.04,-42.2038804065906));
#59425=CARTESIAN_POINT('',(36.312,23.04,-42.2038804065906));
#59426=CARTESIAN_POINT('',(36.1604455912102,23.04,-42.6024987098885));
#59427=CARTESIAN_POINT('Origin',(35.712,23.04,-42.2038804065906));
#59428=CARTESIAN_POINT('Origin',(35.712,23.04,-42.2038804065906));
#59429=CARTESIAN_POINT('Origin',(35.712,23.04,-42.2038804065906));
#59430=CARTESIAN_POINT('Origin',(35.712,23.04,44.6314718625761));
#59431=CARTESIAN_POINT('',(36.312,23.04,44.6314718625761));
#59432=CARTESIAN_POINT('Origin',(35.712,23.04,44.6314718625761));
#59433=CARTESIAN_POINT('',(36.1362640687119,23.04,45.0557359312881));
#59434=CARTESIAN_POINT('Origin',(35.712,23.04,44.6314718625761));
#59435=CARTESIAN_POINT('Origin',(35.712,23.04,44.6314718625761));
#59436=CARTESIAN_POINT('Origin',(35.712,23.04,23.052));
#59437=CARTESIAN_POINT('',(36.312,23.04,23.052));
#59438=CARTESIAN_POINT('Origin',(32.7785603614138,23.04,-45.504));
#59439=CARTESIAN_POINT('',(33.227005952624,23.04,-45.902618303298));
#59440=CARTESIAN_POINT('',(32.7785603614138,23.04,-46.104));
#59441=CARTESIAN_POINT('Origin',(32.7785603614138,23.04,-45.504));
#59442=CARTESIAN_POINT('Origin',(32.7785603614138,23.04,-45.504));
#59443=CARTESIAN_POINT('Origin',(32.7785603614138,23.04,-45.504));
#59444=CARTESIAN_POINT('Origin',(38.6886026846519,23.04,-38.8552023863572));
#59445=CARTESIAN_POINT('',(39.1370482758621,23.04,-39.2538206896552));
#59446=CARTESIAN_POINT('Origin',(-32.7785603614138,23.04,-45.504));
#59447=CARTESIAN_POINT('',(-32.7785603614138,23.04,-46.104));
#59448=CARTESIAN_POINT('',(-33.227005952624,23.04,-45.902618303298));
#59449=CARTESIAN_POINT('Origin',(-32.7785603614138,23.04,-45.504));
#59450=CARTESIAN_POINT('Origin',(-32.7785603614138,23.04,-45.504));
#59451=CARTESIAN_POINT('Origin',(-32.7785603614138,23.04,-45.504));
#59452=CARTESIAN_POINT('Origin',(16.524,23.04,-45.504));
#59453=CARTESIAN_POINT('',(16.524,23.04,-46.104));
#59454=CARTESIAN_POINT('Origin',(-37.0566026846519,23.04,-40.6912023863572));
#59455=CARTESIAN_POINT('',(-36.1604455912102,23.04,-42.6024987098885));
#59456=CARTESIAN_POINT('Origin',(-35.712,23.04,-42.2038804065906));
#59457=CARTESIAN_POINT('',(-37.5050482758621,23.04,-41.0898206896552));
#59458=CARTESIAN_POINT('Origin',(-35.712,23.04,-42.2038804065906));
#59459=CARTESIAN_POINT('',(-36.312,23.04,-42.2038804065906));
#59460=CARTESIAN_POINT('Origin',(-35.712,23.04,-42.2038804065906));
#59461=CARTESIAN_POINT('Origin',(-35.712,23.04,-42.2038804065906));
#59462=CARTESIAN_POINT('Origin',(-32.7785603614138,22.44,-45.504));
#59463=CARTESIAN_POINT('',(-33.227005952624,25.104,-45.902618303298));
#59464=CARTESIAN_POINT('',(-32.7785603614138,25.104,-46.104));
#59465=CARTESIAN_POINT('Origin',(-32.7785603614138,25.104,-45.504));
#59466=CARTESIAN_POINT('',(-32.7785603614138,22.44,-46.104));
#59467=CARTESIAN_POINT('',(-33.227005952624,22.44,-45.902618303298));
#59468=CARTESIAN_POINT('Origin',(-32.7785603614138,25.104,-45.504));
#59469=CARTESIAN_POINT('',(-32.7785603614138,25.704,-45.504));
#59470=CARTESIAN_POINT('Origin',(-32.7785603614138,25.104,-45.504));
#59471=CARTESIAN_POINT('Origin',(-32.7785603614138,25.104,-45.504));
#59472=CARTESIAN_POINT('Origin',(32.7785603614138,22.44,-45.504));
#59473=CARTESIAN_POINT('',(32.7785603614138,25.104,-46.104));
#59474=CARTESIAN_POINT('',(33.227005952624,25.104,-45.902618303298));
#59475=CARTESIAN_POINT('Origin',(32.7785603614138,25.104,-45.504));
#59476=CARTESIAN_POINT('',(33.227005952624,22.44,-45.902618303298));
#59477=CARTESIAN_POINT('',(32.7785603614138,22.44,-46.104));
#59478=CARTESIAN_POINT('Origin',(32.7785603614138,25.104,-45.504));
#59479=CARTESIAN_POINT('',(32.7785603614138,25.704,-45.504));
#59480=CARTESIAN_POINT('Origin',(32.7785603614138,25.104,-45.504));
#59481=CARTESIAN_POINT('Origin',(32.7785603614138,25.104,-45.504));
#59482=CARTESIAN_POINT('Origin',(35.712,22.44,-42.2038804065906));
#59483=CARTESIAN_POINT('',(36.1604455912102,25.104,-42.6024987098885));
#59484=CARTESIAN_POINT('',(36.312,25.104,-42.2038804065906));
#59485=CARTESIAN_POINT('Origin',(35.712,25.104,-42.2038804065906));
#59486=CARTESIAN_POINT('',(36.312,22.44,-42.2038804065906));
#59487=CARTESIAN_POINT('',(36.1604455912102,22.44,-42.6024987098885));
#59488=CARTESIAN_POINT('Origin',(35.712,25.104,-42.2038804065906));
#59489=CARTESIAN_POINT('',(35.712,25.704,-42.2038804065906));
#59490=CARTESIAN_POINT('Origin',(35.712,25.104,-42.2038804065906));
#59491=CARTESIAN_POINT('Origin',(35.712,25.104,-42.2038804065906));
#59492=CARTESIAN_POINT('Origin',(36.312,22.44,-42.432));
#59493=CARTESIAN_POINT('',(39.1370482758621,25.104,-39.2538206896552));
#59494=CARTESIAN_POINT('Origin',(33.048,22.44,-46.104));
#59495=CARTESIAN_POINT('',(16.524,25.104,-46.104));
#59496=CARTESIAN_POINT('Origin',(16.524,25.104,-45.504));
#59497=CARTESIAN_POINT('',(16.524,25.704,-45.504));
#59498=CARTESIAN_POINT('Origin',(-37.0566026846519,25.104,-40.6912023863572));
#59499=CARTESIAN_POINT('',(-36.1604455912102,25.104,-42.6024987098885));
#59500=CARTESIAN_POINT('',(-37.5050482758621,25.104,-41.0898206896552));
#59501=CARTESIAN_POINT('',(-35.712,25.704,-42.2038804065906));
#59502=CARTESIAN_POINT('Origin',(-35.712,25.104,-42.2038804065906));
#59503=CARTESIAN_POINT('',(-37.0566026846519,25.704,-40.6912023863572));
#59504=CARTESIAN_POINT('Origin',(-33.048,22.44,-46.104));
#59505=CARTESIAN_POINT('',(-36.1604455912102,22.44,-42.6024987098885));
#59506=CARTESIAN_POINT('Origin',(-29.16,23.04,6.82615721505037));
#59507=CARTESIAN_POINT('',(-28.56,23.04,6.82615721505037));
#59508=CARTESIAN_POINT('Origin',(-29.16,23.04,6.82615721505037));
#59509=CARTESIAN_POINT('',(-28.9987096774194,23.04,7.40407194218737));
#59510=CARTESIAN_POINT('Origin',(-29.16,23.04,6.82615721505037));
#59511=CARTESIAN_POINT('Origin',(-29.16,23.04,6.82615721505037));
#59512=CARTESIAN_POINT('Origin',(-29.16,25.104,6.82615721505037));
#59513=CARTESIAN_POINT('',(-28.9987096774194,25.104,7.40407194218737));
#59514=CARTESIAN_POINT('',(-28.56,25.104,6.82615721505037));
#59515=CARTESIAN_POINT('Origin',(-29.16,25.104,6.82615721505037));
#59516=CARTESIAN_POINT('',(-29.16,25.704,6.82615721505037));
#59517=CARTESIAN_POINT('Origin',(-29.16,25.104,6.82615721505037));
#59518=CARTESIAN_POINT('Origin',(-29.16,25.104,6.82615721505037));
#59519=CARTESIAN_POINT('Origin',(-29.16,22.44,6.82615721505037));
#59520=CARTESIAN_POINT('',(-28.9987096774194,22.44,7.40407194218737));
#59521=CARTESIAN_POINT('',(-28.56,22.44,6.82615721505037));
#59522=CARTESIAN_POINT('Origin',(-28.56,23.04,8.976));
#59523=CARTESIAN_POINT('',(-26.9880719421874,23.04,9.41470967741935));
#59524=CARTESIAN_POINT('Origin',(-26.4101572150504,23.04,9.576));
#59525=CARTESIAN_POINT('Origin',(-28.56,23.04,8.976));
#59526=CARTESIAN_POINT('Origin',(-26.4101572150504,23.04,9.576));
#59527=CARTESIAN_POINT('',(-26.4101572150504,23.04,8.976));
#59528=CARTESIAN_POINT('Origin',(-26.4101572150504,23.04,9.576));
#59529=CARTESIAN_POINT('Origin',(-26.4101572150504,23.04,9.576));
#59530=CARTESIAN_POINT('Origin',(-29.16,23.04,-16.932));
#59531=CARTESIAN_POINT('',(-28.56,23.04,-32.9381572150504));
#59532=CARTESIAN_POINT('Origin',(-29.16,23.04,-32.9381572150504));
#59533=CARTESIAN_POINT('',(-28.56,23.04,-16.932));
#59534=CARTESIAN_POINT('Origin',(-28.56,23.04,-35.088));
#59535=CARTESIAN_POINT('',(-28.9987096774194,23.04,-33.5160719421874));
#59536=CARTESIAN_POINT('Origin',(-28.56,23.04,-35.088));
#59537=CARTESIAN_POINT('Origin',(-29.16,23.04,-32.9381572150504));
#59538=CARTESIAN_POINT('Origin',(-8.976,23.04,-35.688));
#59539=CARTESIAN_POINT('Origin',(-17.952,23.04,-35.088));
#59540=CARTESIAN_POINT('Origin',(-17.352,23.04,5.1));
#59541=CARTESIAN_POINT('Origin',(-20.1018427849496,23.04,9.576));
#59542=CARTESIAN_POINT('Origin',(-20.1018427849496,23.04,9.576));
#59543=CARTESIAN_POINT('',(-20.1018427849496,23.04,8.976));
#59544=CARTESIAN_POINT('Origin',(-20.1018427849496,23.04,9.576));
#59545=CARTESIAN_POINT('Origin',(-20.1018427849496,23.04,9.576));
#59546=CARTESIAN_POINT('Origin',(-17.952,23.04,8.976));
#59547=CARTESIAN_POINT('Origin',(-29.16,23.04,-32.9381572150504));
#59548=CARTESIAN_POINT('Origin',(-29.16,23.04,-32.9381572150504));
#59549=CARTESIAN_POINT('Origin',(-28.56,25.104,8.976));
#59550=CARTESIAN_POINT('',(-26.4101572150504,25.704,9.576));
#59551=CARTESIAN_POINT('Origin',(-28.56,25.704,8.976));
#59552=CARTESIAN_POINT('',(-26.9880719421874,25.104,9.41470967741935));
#59553=CARTESIAN_POINT('Origin',(-26.4101572150504,25.104,9.576));
#59554=CARTESIAN_POINT('Origin',(-28.56,25.104,8.976));
#59555=CARTESIAN_POINT('Origin',(-29.16,25.104,-16.932));
#59556=CARTESIAN_POINT('',(-28.56,25.104,-32.9381572150504));
#59557=CARTESIAN_POINT('',(-28.56,25.104,-16.932));
#59558=CARTESIAN_POINT('Origin',(-29.16,25.104,-32.9381572150504));
#59559=CARTESIAN_POINT('',(-29.16,25.704,-16.932));
#59560=CARTESIAN_POINT('Origin',(-28.56,22.44,-35.088));
#59561=CARTESIAN_POINT('',(-28.56,22.44,-32.9381572150504));
#59562=CARTESIAN_POINT('Origin',(-29.16,22.44,-32.9381572150504));
#59563=CARTESIAN_POINT('',(-28.9987096774194,22.44,-33.5160719421874));
#59564=CARTESIAN_POINT('Origin',(-29.16,25.104,-32.9381572150504));
#59565=CARTESIAN_POINT('Origin',(-28.56,22.44,-35.088));
#59566=CARTESIAN_POINT('Origin',(-20.1018427849496,22.44,9.576));
#59567=CARTESIAN_POINT('',(-20.1018427849496,25.104,8.976));
#59568=CARTESIAN_POINT('',(-20.1018427849496,22.44,8.976));
#59569=CARTESIAN_POINT('Origin',(-20.1018427849496,25.104,9.576));
#59570=CARTESIAN_POINT('Origin',(28.152,23.04,28.56));
#59571=CARTESIAN_POINT('',(28.152,23.04,26.06));
#59572=CARTESIAN_POINT('Origin',(28.152,23.04,25.46));
#59573=CARTESIAN_POINT('',(25.652,23.04,28.56));
#59574=CARTESIAN_POINT('Origin',(28.152,23.04,28.56));
#59575=CARTESIAN_POINT('Origin',(28.152,23.04,28.56));
#59576=CARTESIAN_POINT('Origin',(28.152,22.44,28.56));
#59577=CARTESIAN_POINT('',(25.652,25.104,28.56));
#59578=CARTESIAN_POINT('',(25.652,22.44,28.56));
#59579=CARTESIAN_POINT('',(28.152,25.104,31.06));
#59580=CARTESIAN_POINT('Origin',(28.152,25.104,28.56));
#59581=CARTESIAN_POINT('Origin',(28.152,25.104,28.56));
#59582=CARTESIAN_POINT('Origin',(-35.712,23.04,44.6314718625761));
#59583=CARTESIAN_POINT('',(-36.312,23.04,44.6314718625761));
#59584=CARTESIAN_POINT('',(-36.1362640687119,23.04,45.0557359312881));
#59585=CARTESIAN_POINT('Origin',(-35.712,23.04,44.6314718625761));
#59586=CARTESIAN_POINT('Origin',(-35.712,23.04,44.6314718625761));
#59587=CARTESIAN_POINT('Origin',(-35.712,23.04,44.6314718625761));
#59588=CARTESIAN_POINT('Origin',(-35.712,23.04,-20.604));
#59589=CARTESIAN_POINT('',(-36.312,23.04,-20.604));
#59590=CARTESIAN_POINT('Origin',(-32.3914718625761,23.04,47.952));
#59591=CARTESIAN_POINT('',(-32.8157359312881,23.04,48.3762640687119));
#59592=CARTESIAN_POINT('',(-32.3914718625761,23.04,48.552));
#59593=CARTESIAN_POINT('Origin',(-32.3914718625761,23.04,47.952));
#59594=CARTESIAN_POINT('Origin',(-32.3914718625761,23.04,47.952));
#59595=CARTESIAN_POINT('Origin',(-32.3914718625761,23.04,47.952));
#59596=CARTESIAN_POINT('Origin',(-37.7237359312881,23.04,42.619735931288));
#59597=CARTESIAN_POINT('',(-38.148,23.04,43.044));
#59598=CARTESIAN_POINT('Origin',(-14.472,23.04,47.952));
#59599=CARTESIAN_POINT('',(-14.472,23.04,48.552));
#59600=CARTESIAN_POINT('',(-13.872,23.04,47.952));
#59601=CARTESIAN_POINT('Origin',(-14.472,23.04,47.952));
#59602=CARTESIAN_POINT('Origin',(-14.472,23.04,47.952));
#59603=CARTESIAN_POINT('Origin',(-14.472,23.04,47.952));
#59604=CARTESIAN_POINT('Origin',(-16.32,23.04,47.952));
#59605=CARTESIAN_POINT('',(-16.32,23.04,48.552));
#59606=CARTESIAN_POINT('Origin',(-14.472,23.04,39.768));
#59607=CARTESIAN_POINT('',(-13.872,23.04,39.768));
#59608=CARTESIAN_POINT('',(-14.472,23.04,39.168));
#59609=CARTESIAN_POINT('Origin',(-14.472,23.04,39.768));
#59610=CARTESIAN_POINT('Origin',(-14.472,23.04,39.768));
#59611=CARTESIAN_POINT('Origin',(-14.472,23.04,39.768));
#59612=CARTESIAN_POINT('Origin',(-14.472,23.04,24.888));
#59613=CARTESIAN_POINT('',(-13.872,23.04,24.888));
#59614=CARTESIAN_POINT('Origin',(-6.936,23.04,39.768));
#59615=CARTESIAN_POINT('',(-16.728,23.04,39.168));
#59616=CARTESIAN_POINT('',(-6.936,23.04,39.168));
#59617=CARTESIAN_POINT('Origin',(-17.328,23.04,39.768));
#59618=CARTESIAN_POINT('Origin',(-17.328,23.04,20.196));
#59619=CARTESIAN_POINT('',(-16.728,23.04,33.048));
#59620=CARTESIAN_POINT('Origin',(-17.328,23.04,32.448));
#59621=CARTESIAN_POINT('',(-16.728,23.04,20.196));
#59622=CARTESIAN_POINT('Origin',(-14.472,23.04,32.448));
#59623=CARTESIAN_POINT('',(-14.472,23.04,33.048));
#59624=CARTESIAN_POINT('',(-13.872,23.04,32.448));
#59625=CARTESIAN_POINT('Origin',(-14.472,23.04,32.448));
#59626=CARTESIAN_POINT('Origin',(-14.472,23.04,32.448));
#59627=CARTESIAN_POINT('Origin',(-14.472,23.04,32.448));
#59628=CARTESIAN_POINT('Origin',(-8.364,23.04,32.448));
#59629=CARTESIAN_POINT('',(-8.364,23.04,33.048));
#59630=CARTESIAN_POINT('Origin',(-14.472,23.04,17.136));
#59631=CARTESIAN_POINT('',(-13.872,23.04,17.136));
#59632=CARTESIAN_POINT('Origin',(-14.472,22.44,32.448));
#59633=CARTESIAN_POINT('',(-13.872,25.104,32.448));
#59634=CARTESIAN_POINT('',(-14.472,25.104,33.048));
#59635=CARTESIAN_POINT('Origin',(-14.472,25.104,32.448));
#59636=CARTESIAN_POINT('',(-14.472,22.44,33.048));
#59637=CARTESIAN_POINT('',(-13.872,22.44,32.448));
#59638=CARTESIAN_POINT('Origin',(-14.472,25.104,32.448));
#59639=CARTESIAN_POINT('',(-14.472,25.704,32.448));
#59640=CARTESIAN_POINT('Origin',(-14.472,25.104,32.448));
#59641=CARTESIAN_POINT('Origin',(-14.472,25.104,32.448));
#59642=CARTESIAN_POINT('Origin',(-14.472,22.44,39.768));
#59643=CARTESIAN_POINT('',(-14.472,25.104,39.168));
#59644=CARTESIAN_POINT('',(-13.872,25.104,39.768));
#59645=CARTESIAN_POINT('Origin',(-14.472,25.104,39.768));
#59646=CARTESIAN_POINT('',(-13.872,22.44,39.768));
#59647=CARTESIAN_POINT('',(-14.472,22.44,39.168));
#59648=CARTESIAN_POINT('Origin',(-14.472,25.104,39.768));
#59649=CARTESIAN_POINT('',(-14.472,25.704,39.768));
#59650=CARTESIAN_POINT('Origin',(-14.472,25.104,39.768));
#59651=CARTESIAN_POINT('Origin',(-14.472,25.104,39.768));
#59652=CARTESIAN_POINT('Origin',(-14.472,22.44,47.952));
#59653=CARTESIAN_POINT('',(-13.872,25.104,47.952));
#59654=CARTESIAN_POINT('',(-14.472,25.104,48.552));
#59655=CARTESIAN_POINT('Origin',(-14.472,25.104,47.952));
#59656=CARTESIAN_POINT('',(-14.472,22.44,48.552));
#59657=CARTESIAN_POINT('',(-13.872,22.44,47.952));
#59658=CARTESIAN_POINT('Origin',(-14.472,25.104,47.952));
#59659=CARTESIAN_POINT('',(-14.472,25.704,47.952));
#59660=CARTESIAN_POINT('Origin',(-14.472,25.104,47.952));
#59661=CARTESIAN_POINT('Origin',(-14.472,25.104,47.952));
#59662=CARTESIAN_POINT('Origin',(-32.3914718625761,22.44,47.952));
#59663=CARTESIAN_POINT('',(-32.3914718625761,25.104,48.552));
#59664=CARTESIAN_POINT('',(-32.8157359312881,25.104,48.3762640687119));
#59665=CARTESIAN_POINT('Origin',(-32.3914718625761,25.104,47.952));
#59666=CARTESIAN_POINT('',(-32.8157359312881,22.44,48.3762640687119));
#59667=CARTESIAN_POINT('',(-32.3914718625761,22.44,48.552));
#59668=CARTESIAN_POINT('Origin',(-32.3914718625761,25.104,47.952));
#59669=CARTESIAN_POINT('',(-32.3914718625761,25.704,47.952));
#59670=CARTESIAN_POINT('Origin',(-32.3914718625761,25.104,47.952));
#59671=CARTESIAN_POINT('Origin',(-32.3914718625761,25.104,47.952));
#59672=CARTESIAN_POINT('Origin',(-35.712,22.44,44.6314718625761));
#59673=CARTESIAN_POINT('',(-36.1362640687119,25.104,45.0557359312881));
#59674=CARTESIAN_POINT('',(-36.312,25.104,44.6314718625761));
#59675=CARTESIAN_POINT('Origin',(-35.712,25.104,44.6314718625761));
#59676=CARTESIAN_POINT('',(-36.312,22.44,44.6314718625761));
#59677=CARTESIAN_POINT('',(-36.1362640687119,22.44,45.0557359312881));
#59678=CARTESIAN_POINT('Origin',(-35.712,25.104,44.6314718625761));
#59679=CARTESIAN_POINT('',(-35.712,25.704,44.6314718625761));
#59680=CARTESIAN_POINT('Origin',(-35.712,25.104,44.6314718625761));
#59681=CARTESIAN_POINT('Origin',(-35.712,25.104,44.6314718625761));
#59682=CARTESIAN_POINT('Origin',(-35.712,22.44,-42.2038804065906));
#59683=CARTESIAN_POINT('',(-36.312,25.104,-42.2038804065906));
#59684=CARTESIAN_POINT('',(-36.312,22.44,-42.2038804065906));
#59685=CARTESIAN_POINT('Origin',(-35.712,25.104,-42.2038804065906));
#59686=CARTESIAN_POINT('Origin',(-35.712,25.104,-42.2038804065906));
#59687=CARTESIAN_POINT('Origin',(-35.712,25.104,-42.2038804065906));
#59688=CARTESIAN_POINT('Origin',(-32.64,22.44,48.552));
#59689=CARTESIAN_POINT('',(-16.32,25.104,48.552));
#59690=CARTESIAN_POINT('Origin',(-37.7237359312881,25.104,42.619735931288));
#59691=CARTESIAN_POINT('',(-37.7237359312881,25.704,42.619735931288));
#59692=CARTESIAN_POINT('',(-38.148,25.104,43.044));
#59693=CARTESIAN_POINT('Origin',(-16.32,25.104,47.952));
#59694=CARTESIAN_POINT('',(-16.32,25.704,47.952));
#59695=CARTESIAN_POINT('Origin',(-13.872,22.44,48.552));
#59696=CARTESIAN_POINT('',(-13.872,25.104,24.888));
#59697=CARTESIAN_POINT('Origin',(-14.472,25.104,24.888));
#59698=CARTESIAN_POINT('',(-14.472,25.704,24.888));
#59699=CARTESIAN_POINT('Origin',(-6.936,25.104,39.768));
#59700=CARTESIAN_POINT('',(-16.728,25.104,39.168));
#59701=CARTESIAN_POINT('',(-6.936,25.104,39.168));
#59702=CARTESIAN_POINT('',(-17.328,25.704,39.768));
#59703=CARTESIAN_POINT('Origin',(-17.328,25.104,39.768));
#59704=CARTESIAN_POINT('',(-6.936,25.704,39.768));
#59705=CARTESIAN_POINT('Origin',(-13.872,22.44,39.168));
#59706=CARTESIAN_POINT('',(-16.728,22.44,39.168));
#59707=CARTESIAN_POINT('Origin',(-16.728,22.44,39.168));
#59708=CARTESIAN_POINT('',(-16.728,25.104,33.048));
#59709=CARTESIAN_POINT('',(-16.728,22.44,33.048));
#59710=CARTESIAN_POINT('',(-16.728,25.104,20.196));
#59711=CARTESIAN_POINT('Origin',(-16.728,22.44,33.048));
#59712=CARTESIAN_POINT('',(-8.364,25.104,33.048));
#59713=CARTESIAN_POINT('Origin',(-8.364,25.104,32.448));
#59714=CARTESIAN_POINT('',(-17.328,25.704,32.448));
#59715=CARTESIAN_POINT('',(-8.364,25.704,32.448));
#59716=CARTESIAN_POINT('Origin',(-17.328,25.104,32.448));
#59717=CARTESIAN_POINT('Origin',(-14.472,25.104,17.136));
#59718=CARTESIAN_POINT('',(-13.872,25.104,13.056));
#59719=CARTESIAN_POINT('',(-13.872,25.104,17.136));
#59720=CARTESIAN_POINT('',(-14.472,25.704,12.8074718625761));
#59721=CARTESIAN_POINT('Origin',(-14.472,25.104,12.8074718625761));
#59722=CARTESIAN_POINT('',(-14.472,25.704,17.136));
#59723=CARTESIAN_POINT('Origin',(-13.872,22.44,33.048));
#59724=CARTESIAN_POINT('',(-13.872,22.44,13.056));
#59725=CARTESIAN_POINT('Origin',(28.152,25.104,28.56));
#59726=CARTESIAN_POINT('',(28.152,25.704,31.66));
#59727=CARTESIAN_POINT('Origin',(28.152,25.704,28.56));
#59728=CARTESIAN_POINT('Origin',(28.152,25.104,31.66));
#59729=CARTESIAN_POINT('Origin',(0.,25.704,1.224));
#59730=CARTESIAN_POINT('',(-8.1888,25.704,6.52427186257614));
#59731=CARTESIAN_POINT('',(-7.87026406871193,25.704,6.20573593128807));
#59732=CARTESIAN_POINT('',(-8.1888,25.704,-21.7872));
#59733=CARTESIAN_POINT('',(-8.1888,25.704,3.9984));
#59734=CARTESIAN_POINT('',(8.1888,25.704,-21.7872));
#59735=CARTESIAN_POINT('Origin',(0.,25.704,-21.7872));
#59736=CARTESIAN_POINT('',(8.1888,25.704,6.52427186257614));
#59737=CARTESIAN_POINT('',(8.1888,25.704,-10.2816));
#59738=CARTESIAN_POINT('',(14.472,25.704,12.8074718625761));
#59739=CARTESIAN_POINT('',(4.72866406871193,25.704,3.06413593128807));
#59740=CARTESIAN_POINT('',(14.472,25.704,32.448));
#59741=CARTESIAN_POINT('',(14.472,25.704,7.14));
#59742=CARTESIAN_POINT('',(17.328,25.704,32.448));
#59743=CARTESIAN_POINT('',(6.936,25.704,32.448));
#59744=CARTESIAN_POINT('',(17.328,25.704,39.768));
#59745=CARTESIAN_POINT('',(17.328,25.704,17.136));
#59746=CARTESIAN_POINT('',(14.472,25.704,39.768));
#59747=CARTESIAN_POINT('',(8.364,25.704,39.768));
#59748=CARTESIAN_POINT('',(14.472,25.704,47.952));
#59749=CARTESIAN_POINT('',(14.472,25.704,20.196));
#59750=CARTESIAN_POINT('',(32.3914718625761,25.704,47.952));
#59751=CARTESIAN_POINT('',(6.936,25.704,47.952));
#59752=CARTESIAN_POINT('',(35.712,25.704,44.6314718625761));
#59753=CARTESIAN_POINT('',(35.8877359312881,25.704,44.455735931288));
#59754=CARTESIAN_POINT('',(35.712,25.704,23.052));
#59755=CARTESIAN_POINT('',(38.6886026846519,25.704,-38.8552023863572));
#59756=CARTESIAN_POINT('',(-35.712,25.704,-20.604));
#59757=CARTESIAN_POINT('',(-17.328,25.704,20.196));
#59758=CARTESIAN_POINT('',(17.352,25.704,6.82615721505037));
#59759=CARTESIAN_POINT('Origin',(17.952,25.704,8.976));
#59760=CARTESIAN_POINT('',(17.352,25.704,-32.9381572150504));
#59761=CARTESIAN_POINT('',(17.352,25.704,-16.932));
#59762=CARTESIAN_POINT('',(20.1018427849496,25.704,-35.688));
#59763=CARTESIAN_POINT('Origin',(17.952,25.704,-35.088));
#59764=CARTESIAN_POINT('',(26.4101572150504,25.704,-35.688));
#59765=CARTESIAN_POINT('',(14.28,25.704,-35.688));
#59766=CARTESIAN_POINT('Origin',(28.56,25.704,-35.088));
#59767=CARTESIAN_POINT('',(3.456,25.704,-35.496));
#59768=CARTESIAN_POINT('',(3.456,25.704,-37.944));
#59769=CARTESIAN_POINT('',(3.456,25.704,-17.136));
#59770=CARTESIAN_POINT('',(-3.456,25.704,-35.496));
#59771=CARTESIAN_POINT('Origin',(0.,25.704,-35.496));
#59772=CARTESIAN_POINT('',(-3.456,25.704,-37.944));
#59773=CARTESIAN_POINT('',(-3.456,25.704,-18.36));
#59774=CARTESIAN_POINT('Origin',(0.,25.704,-37.944));
#59775=CARTESIAN_POINT('',(29.376,25.704,33.6154718625761));
#59776=CARTESIAN_POINT('Origin',(29.376,25.704,38.352));
#59777=CARTESIAN_POINT('',(-14.28,25.704,9.576));
#59778=CARTESIAN_POINT('',(-29.376,25.704,33.6154718625761));
#59779=CARTESIAN_POINT('Origin',(-29.376,25.704,38.352));
#59780=CARTESIAN_POINT('',(-28.152,25.704,31.66));
#59781=CARTESIAN_POINT('Origin',(-28.152,25.704,28.56));
#59782=CARTESIAN_POINT('Origin',(-20.1018427849496,25.104,9.576));
#59783=CARTESIAN_POINT('Origin',(-20.1018427849496,25.104,9.576));
#59784=CARTESIAN_POINT('Origin',(-14.28,25.104,9.576));
#59785=CARTESIAN_POINT('',(-26.4101572150504,25.104,8.976));
#59786=CARTESIAN_POINT('Origin',(-26.4101572150504,25.104,9.576));
#59787=CARTESIAN_POINT('',(-14.28,25.104,8.976));
#59788=CARTESIAN_POINT('Origin',(-14.28,23.04,9.576));
#59789=CARTESIAN_POINT('',(-14.28,23.04,8.976));
#59790=CARTESIAN_POINT('Origin',(-26.4101572150504,22.44,9.576));
#59791=CARTESIAN_POINT('',(-26.9880719421874,22.44,9.41470967741935));
#59792=CARTESIAN_POINT('Origin',(-26.4101572150504,25.104,9.576));
#59793=CARTESIAN_POINT('',(-26.4101572150504,22.44,8.976));
#59794=CARTESIAN_POINT('Origin',(-26.4101572150504,25.104,9.576));
#59795=CARTESIAN_POINT('Origin',(-29.16,25.104,-32.9381572150504));
#59796=CARTESIAN_POINT('Origin',(-28.56,22.44,8.976));
#59797=CARTESIAN_POINT('Origin',(-28.56,22.44,8.976));
#59798=CARTESIAN_POINT('Origin',(-17.328,25.104,20.196));
#59799=CARTESIAN_POINT('Origin',(-35.712,25.104,-20.604));
#59800=CARTESIAN_POINT('',(-36.312,25.104,-20.604));
#59801=CARTESIAN_POINT('Origin',(38.6886026846519,25.104,-38.8552023863572));
#59802=CARTESIAN_POINT('Origin',(35.712,25.104,44.6314718625761));
#59803=CARTESIAN_POINT('',(36.312,25.104,44.6314718625761));
#59804=CARTESIAN_POINT('Origin',(35.712,25.104,44.6314718625761));
#59805=CARTESIAN_POINT('',(36.1362640687119,25.104,45.0557359312881));
#59806=CARTESIAN_POINT('Origin',(35.712,25.104,44.6314718625761));
#59807=CARTESIAN_POINT('Origin',(35.712,25.104,44.6314718625761));
#59808=CARTESIAN_POINT('Origin',(35.712,25.104,23.052));
#59809=CARTESIAN_POINT('',(36.312,25.104,23.052));
#59810=CARTESIAN_POINT('Origin',(-36.312,22.44,44.88));
#59811=CARTESIAN_POINT('Origin',(-36.312,22.44,-42.432));
#59812=CARTESIAN_POINT('Origin',(36.312,22.44,44.88));
#59813=CARTESIAN_POINT('',(36.312,22.44,44.6314718625761));
#59814=CARTESIAN_POINT('Origin',(35.712,22.44,44.6314718625761));
#59815=CARTESIAN_POINT('',(36.1362640687119,22.44,45.0557359312881));
#59816=CARTESIAN_POINT('Origin',(17.352,23.04,6.82615721505037));
#59817=CARTESIAN_POINT('',(17.952,23.04,6.82615721505037));
#59818=CARTESIAN_POINT('Origin',(17.352,23.04,6.82615721505037));
#59819=CARTESIAN_POINT('Origin',(17.352,23.04,6.82615721505036));
#59820=CARTESIAN_POINT('Origin',(17.352,23.04,-32.9381572150504));
#59821=CARTESIAN_POINT('',(17.952,23.04,-32.9381572150504));
#59822=CARTESIAN_POINT('',(17.5132903225806,23.04,-33.5160719421874));
#59823=CARTESIAN_POINT('Origin',(17.352,23.04,-32.9381572150504));
#59824=CARTESIAN_POINT('Origin',(17.352,23.04,-32.9381572150504));
#59825=CARTESIAN_POINT('Origin',(17.352,23.04,-32.9381572150504));
#59826=CARTESIAN_POINT('Origin',(17.352,23.04,-16.932));
#59827=CARTESIAN_POINT('',(17.952,23.04,-16.932));
#59828=CARTESIAN_POINT('Origin',(20.1018427849496,23.04,-35.688));
#59829=CARTESIAN_POINT('',(19.5239280578126,23.04,-35.5267096774194));
#59830=CARTESIAN_POINT('Origin',(20.1018427849496,23.04,-35.688));
#59831=CARTESIAN_POINT('',(20.1018427849496,23.04,-35.088));
#59832=CARTESIAN_POINT('Origin',(20.1018427849496,23.04,-35.688));
#59833=CARTESIAN_POINT('Origin',(20.1018427849496,23.04,-35.688));
#59834=CARTESIAN_POINT('Origin',(17.952,23.04,-35.088));
#59835=CARTESIAN_POINT('Origin',(17.952,23.04,-35.088));
#59836=CARTESIAN_POINT('Origin',(17.352,22.44,-32.9381572150504));
#59837=CARTESIAN_POINT('',(17.5132903225806,25.104,-33.5160719421874));
#59838=CARTESIAN_POINT('',(17.952,25.104,-32.9381572150504));
#59839=CARTESIAN_POINT('Origin',(17.352,25.104,-32.9381572150504));
#59840=CARTESIAN_POINT('',(17.952,22.44,-32.9381572150504));
#59841=CARTESIAN_POINT('',(17.5132903225806,22.44,-33.5160719421874));
#59842=CARTESIAN_POINT('Origin',(17.352,25.104,-32.9381572150504));
#59843=CARTESIAN_POINT('Origin',(17.352,25.104,-32.9381572150504));
#59844=CARTESIAN_POINT('Origin',(17.352,25.104,-32.9381572150504));
#59845=CARTESIAN_POINT('Origin',(17.352,25.104,6.82615721505037));
#59846=CARTESIAN_POINT('',(17.5132903225806,25.104,7.40407194218736));
#59847=CARTESIAN_POINT('',(17.952,25.104,6.82615721505036));
#59848=CARTESIAN_POINT('Origin',(17.352,25.104,6.82615721505037));
#59849=CARTESIAN_POINT('Origin',(17.352,25.104,6.82615721505036));
#59850=CARTESIAN_POINT('Origin',(17.352,25.104,6.82615721505037));
#59851=CARTESIAN_POINT('Origin',(17.352,22.44,6.82615721505037));
#59852=CARTESIAN_POINT('',(17.5132903225806,22.44,7.40407194218736));
#59853=CARTESIAN_POINT('',(17.952,22.44,6.82615721505037));
#59854=CARTESIAN_POINT('Origin',(20.1018427849496,25.104,9.576));
#59855=CARTESIAN_POINT('Origin',(20.1018427849496,25.104,9.576));
#59856=CARTESIAN_POINT('Origin',(17.952,22.44,8.976));
#59857=CARTESIAN_POINT('Origin',(17.952,25.104,8.976));
#59858=CARTESIAN_POINT('Origin',(17.952,25.104,8.976));
#59859=CARTESIAN_POINT('Origin',(29.16,25.104,-32.9381572150504));
#59860=CARTESIAN_POINT('',(28.9987096774194,25.104,-33.5160719421874));
#59861=CARTESIAN_POINT('Origin',(29.16,25.104,-32.9381572150504));
#59862=CARTESIAN_POINT('Origin',(29.16,25.104,-32.9381572150504));
#59863=CARTESIAN_POINT('Origin',(29.16,22.44,-32.9381572150504));
#59864=CARTESIAN_POINT('',(28.9987096774193,22.44,-33.5160719421874));
#59865=CARTESIAN_POINT('Origin',(28.56,23.04,-35.088));
#59866=CARTESIAN_POINT('',(26.9880719421874,23.04,-35.5267096774194));
#59867=CARTESIAN_POINT('Origin',(28.56,23.04,-35.088));
#59868=CARTESIAN_POINT('Origin',(26.4101572150504,23.04,-35.688));
#59869=CARTESIAN_POINT('Origin',(26.4101572150504,23.04,-35.688));
#59870=CARTESIAN_POINT('',(26.4101572150504,23.04,-35.088));
#59871=CARTESIAN_POINT('Origin',(26.4101572150504,23.04,-35.688));
#59872=CARTESIAN_POINT('Origin',(26.4101572150504,23.04,-35.688));
#59873=CARTESIAN_POINT('Origin',(28.56,25.104,-35.088));
#59874=CARTESIAN_POINT('',(26.9880719421874,25.104,-35.5267096774194));
#59875=CARTESIAN_POINT('Origin',(26.4101572150504,25.104,-35.688));
#59876=CARTESIAN_POINT('Origin',(28.56,25.104,-35.088));
#59877=CARTESIAN_POINT('Origin',(20.1018427849496,25.104,-35.688));
#59878=CARTESIAN_POINT('',(19.5239280578126,25.104,-35.5267096774194));
#59879=CARTESIAN_POINT('',(20.1018427849496,25.104,-35.088));
#59880=CARTESIAN_POINT('Origin',(20.1018427849496,25.104,-35.688));
#59881=CARTESIAN_POINT('Origin',(20.1018427849496,25.104,-35.688));
#59882=CARTESIAN_POINT('Origin',(20.1018427849496,25.104,-35.688));
#59883=CARTESIAN_POINT('Origin',(20.1018427849496,22.44,-35.688));
#59884=CARTESIAN_POINT('',(20.1018427849496,22.44,-35.088));
#59885=CARTESIAN_POINT('',(19.5239280578126,22.44,-35.5267096774194));
#59886=CARTESIAN_POINT('Origin',(14.28,23.04,-35.688));
#59887=CARTESIAN_POINT('',(14.28,23.04,-35.088));
#59888=CARTESIAN_POINT('Origin',(26.4101572150504,22.44,-35.688));
#59889=CARTESIAN_POINT('',(26.9880719421874,22.44,-35.5267096774194));
#59890=CARTESIAN_POINT('',(26.4101572150504,25.104,-35.088));
#59891=CARTESIAN_POINT('Origin',(26.4101572150504,25.104,-35.688));
#59892=CARTESIAN_POINT('',(26.4101572150504,22.44,-35.088));
#59893=CARTESIAN_POINT('Origin',(26.4101572150504,25.104,-35.688));
#59894=CARTESIAN_POINT('Origin',(26.4101572150504,25.104,-35.688));
#59895=CARTESIAN_POINT('Origin',(28.56,22.44,-35.088));
#59896=CARTESIAN_POINT('',(14.28,25.104,-35.088));
#59897=CARTESIAN_POINT('Origin',(28.56,22.44,-35.088));
#59898=CARTESIAN_POINT('Origin',(-7.87026406871193,25.104,6.20573593128807));
#59899=CARTESIAN_POINT('',(-7.76453593128807,25.104,6.94853593128807));
#59900=CARTESIAN_POINT('Origin',(-8.1888,25.104,6.52427186257614));
#59901=CARTESIAN_POINT('',(-7.446,25.104,6.63));
#59902=CARTESIAN_POINT('Origin',(8.1888,23.04,6.52427186257615));
#59903=CARTESIAN_POINT('',(7.5888,23.04,6.52427186257614));
#59904=CARTESIAN_POINT('',(7.76453593128807,23.04,6.94853593128807));
#59905=CARTESIAN_POINT('Origin',(8.1888,23.04,6.52427186257614));
#59906=CARTESIAN_POINT('Origin',(8.1888,23.04,6.52427186257615));
#59907=CARTESIAN_POINT('Origin',(8.1888,23.04,6.52427186257614));
#59908=CARTESIAN_POINT('Origin',(0.,23.04,-21.7872));
#59909=CARTESIAN_POINT('',(7.5888,23.04,-21.7872));
#59910=CARTESIAN_POINT('Origin',(8.1888,23.04,-21.7872));
#59911=CARTESIAN_POINT('Origin',(0.,23.04,-21.7872));
#59912=CARTESIAN_POINT('Origin',(8.1888,23.04,-10.2816));
#59913=CARTESIAN_POINT('',(7.5888,23.04,-10.2816));
#59914=CARTESIAN_POINT('Origin',(4.72866406871193,23.04,3.06413593128807));
#59915=CARTESIAN_POINT('',(13.872,23.04,13.056));
#59916=CARTESIAN_POINT('',(4.3044,23.04,3.4884));
#59917=CARTESIAN_POINT('Origin',(14.472,23.04,12.8074718625761));
#59918=CARTESIAN_POINT('Origin',(14.472,23.04,32.448));
#59919=CARTESIAN_POINT('',(13.872,23.04,32.448));
#59920=CARTESIAN_POINT('',(14.472,23.04,33.048));
#59921=CARTESIAN_POINT('Origin',(14.472,23.04,32.448));
#59922=CARTESIAN_POINT('Origin',(14.472,23.04,32.448));
#59923=CARTESIAN_POINT('Origin',(14.472,23.04,32.448));
#59924=CARTESIAN_POINT('Origin',(14.472,23.04,7.14));
#59925=CARTESIAN_POINT('',(13.872,23.04,7.14));
#59926=CARTESIAN_POINT('Origin',(6.936,23.04,32.448));
#59927=CARTESIAN_POINT('',(16.728,23.04,33.048));
#59928=CARTESIAN_POINT('',(6.936,23.04,33.048));
#59929=CARTESIAN_POINT('Origin',(17.328,23.04,32.448));
#59930=CARTESIAN_POINT('Origin',(17.328,23.04,17.136));
#59931=CARTESIAN_POINT('',(16.728,23.04,39.168));
#59932=CARTESIAN_POINT('Origin',(17.328,23.04,39.768));
#59933=CARTESIAN_POINT('',(16.728,23.04,17.136));
#59934=CARTESIAN_POINT('Origin',(14.472,23.04,39.768));
#59935=CARTESIAN_POINT('',(14.472,23.04,39.168));
#59936=CARTESIAN_POINT('',(13.872,23.04,39.768));
#59937=CARTESIAN_POINT('Origin',(14.472,23.04,39.768));
#59938=CARTESIAN_POINT('Origin',(14.472,23.04,39.768));
#59939=CARTESIAN_POINT('Origin',(14.472,23.04,39.768));
#59940=CARTESIAN_POINT('Origin',(8.364,23.04,39.768));
#59941=CARTESIAN_POINT('',(8.364,23.04,39.168));
#59942=CARTESIAN_POINT('Origin',(14.472,23.04,47.952));
#59943=CARTESIAN_POINT('',(13.872,23.04,47.952));
#59944=CARTESIAN_POINT('',(14.472,23.04,48.552));
#59945=CARTESIAN_POINT('Origin',(14.472,23.04,47.952));
#59946=CARTESIAN_POINT('Origin',(14.472,23.04,47.952));
#59947=CARTESIAN_POINT('Origin',(14.472,23.04,47.952));
#59948=CARTESIAN_POINT('Origin',(14.472,23.04,20.196));
#59949=CARTESIAN_POINT('',(13.872,23.04,20.196));
#59950=CARTESIAN_POINT('Origin',(32.3914718625761,23.04,47.952));
#59951=CARTESIAN_POINT('',(32.3914718625761,23.04,48.552));
#59952=CARTESIAN_POINT('',(32.8157359312881,23.04,48.3762640687119));
#59953=CARTESIAN_POINT('Origin',(32.3914718625761,23.04,47.952));
#59954=CARTESIAN_POINT('Origin',(32.3914718625761,23.04,47.952));
#59955=CARTESIAN_POINT('Origin',(32.3914718625761,23.04,47.952));
#59956=CARTESIAN_POINT('Origin',(6.936,23.04,47.952));
#59957=CARTESIAN_POINT('',(6.936,23.04,48.552));
#59958=CARTESIAN_POINT('Origin',(35.8877359312881,23.04,44.455735931288));
#59959=CARTESIAN_POINT('',(36.312,23.04,44.88));
#59960=CARTESIAN_POINT('Origin',(32.3914718625761,22.44,47.952));
#59961=CARTESIAN_POINT('',(32.8157359312881,25.104,48.3762640687119));
#59962=CARTESIAN_POINT('',(32.3914718625761,25.104,48.552));
#59963=CARTESIAN_POINT('Origin',(32.3914718625761,25.104,47.952));
#59964=CARTESIAN_POINT('',(32.3914718625761,22.44,48.552));
#59965=CARTESIAN_POINT('',(32.8157359312881,22.44,48.3762640687119));
#59966=CARTESIAN_POINT('Origin',(35.8877359312881,25.104,44.455735931288));
#59967=CARTESIAN_POINT('Origin',(32.3914718625761,25.104,47.952));
#59968=CARTESIAN_POINT('',(36.312,25.104,44.88));
#59969=CARTESIAN_POINT('Origin',(14.472,22.44,47.952));
#59970=CARTESIAN_POINT('',(14.472,25.104,48.552));
#59971=CARTESIAN_POINT('',(13.872,25.104,47.952));
#59972=CARTESIAN_POINT('Origin',(14.472,25.104,47.952));
#59973=CARTESIAN_POINT('',(13.872,22.44,47.952));
#59974=CARTESIAN_POINT('',(14.472,22.44,48.552));
#59975=CARTESIAN_POINT('Origin',(14.472,25.104,47.952));
#59976=CARTESIAN_POINT('Origin',(14.472,25.104,47.952));
#59977=CARTESIAN_POINT('Origin',(14.472,25.104,47.952));
#59978=CARTESIAN_POINT('Origin',(14.472,22.44,39.768));
#59979=CARTESIAN_POINT('',(13.872,25.104,39.768));
#59980=CARTESIAN_POINT('',(14.472,25.104,39.168));
#59981=CARTESIAN_POINT('Origin',(14.472,25.104,39.768));
#59982=CARTESIAN_POINT('',(14.472,22.44,39.168));
#59983=CARTESIAN_POINT('',(13.872,22.44,39.768));
#59984=CARTESIAN_POINT('Origin',(14.472,25.104,39.768));
#59985=CARTESIAN_POINT('Origin',(14.472,25.104,39.768));
#59986=CARTESIAN_POINT('Origin',(14.472,25.104,39.768));
#59987=CARTESIAN_POINT('Origin',(14.472,22.44,32.448));
#59988=CARTESIAN_POINT('',(14.472,25.104,33.048));
#59989=CARTESIAN_POINT('',(13.872,25.104,32.448));
#59990=CARTESIAN_POINT('Origin',(14.472,25.104,32.448));
#59991=CARTESIAN_POINT('',(13.872,22.44,32.448));
#59992=CARTESIAN_POINT('',(14.472,22.44,33.048));
#59993=CARTESIAN_POINT('Origin',(14.472,25.104,32.448));
#59994=CARTESIAN_POINT('Origin',(14.472,25.104,32.448));
#59995=CARTESIAN_POINT('Origin',(14.472,25.104,32.448));
#59996=CARTESIAN_POINT('Origin',(8.1888,22.44,6.52427186257614));
#59997=CARTESIAN_POINT('',(7.76453593128807,25.104,6.94853593128807));
#59998=CARTESIAN_POINT('',(7.5888,25.104,6.52427186257614));
#59999=CARTESIAN_POINT('Origin',(8.1888,25.104,6.52427186257614));
#60000=CARTESIAN_POINT('',(7.5888,22.44,6.52427186257614));
#60001=CARTESIAN_POINT('',(7.76453593128807,22.44,6.94853593128807));
#60002=CARTESIAN_POINT('Origin',(8.1888,25.104,6.52427186257614));
#60003=CARTESIAN_POINT('Origin',(8.1888,25.104,6.52427186257615));
#60004=CARTESIAN_POINT('Origin',(8.1888,25.104,6.52427186257614));
#60005=CARTESIAN_POINT('Origin',(-8.1888,22.44,6.52427186257615));
#60006=CARTESIAN_POINT('',(-7.5888,25.104,6.52427186257615));
#60007=CARTESIAN_POINT('',(-7.5888,22.44,6.52427186257615));
#60008=CARTESIAN_POINT('Origin',(-8.1888,25.104,6.52427186257615));
#60009=CARTESIAN_POINT('',(-7.76453593128807,22.44,6.94853593128807));
#60010=CARTESIAN_POINT('Origin',(32.3914718625761,25.104,47.952));
#60011=CARTESIAN_POINT('Origin',(32.3914718625761,25.104,47.952));
#60012=CARTESIAN_POINT('Origin',(-8.1888,25.104,6.52427186257615));
#60013=CARTESIAN_POINT('Origin',(-8.1888,25.104,6.52427186257615));
#60014=CARTESIAN_POINT('Origin',(8.1888,25.104,-10.2816));
#60015=CARTESIAN_POINT('',(7.5888,25.104,-21.7872));
#60016=CARTESIAN_POINT('Origin',(8.1888,25.104,-21.7872));
#60017=CARTESIAN_POINT('',(7.5888,25.104,-10.2816));
#60018=CARTESIAN_POINT('Origin',(4.72866406871193,25.104,3.06413593128807));
#60019=CARTESIAN_POINT('',(13.872,25.104,13.056));
#60020=CARTESIAN_POINT('',(4.3044,25.104,3.4884));
#60021=CARTESIAN_POINT('Origin',(14.472,25.104,12.8074718625761));
#60022=CARTESIAN_POINT('Origin',(7.5888,22.44,6.7728));
#60023=CARTESIAN_POINT('',(13.872,22.44,13.056));
#60024=CARTESIAN_POINT('Origin',(13.872,22.44,13.056));
#60025=CARTESIAN_POINT('',(13.872,25.104,7.14));
#60026=CARTESIAN_POINT('Origin',(14.472,25.104,7.14));
#60027=CARTESIAN_POINT('Origin',(6.936,25.104,32.448));
#60028=CARTESIAN_POINT('',(16.728,25.104,33.048));
#60029=CARTESIAN_POINT('',(6.936,25.104,33.048));
#60030=CARTESIAN_POINT('Origin',(17.328,25.104,32.448));
#60031=CARTESIAN_POINT('Origin',(13.872,22.44,33.048));
#60032=CARTESIAN_POINT('',(16.728,22.44,33.048));
#60033=CARTESIAN_POINT('Origin',(16.728,22.44,33.048));
#60034=CARTESIAN_POINT('',(16.728,25.104,39.168));
#60035=CARTESIAN_POINT('',(16.728,22.44,39.168));
#60036=CARTESIAN_POINT('',(16.728,25.104,17.136));
#60037=CARTESIAN_POINT('Origin',(16.728,22.44,39.168));
#60038=CARTESIAN_POINT('',(8.364,25.104,39.168));
#60039=CARTESIAN_POINT('Origin',(8.364,25.104,39.768));
#60040=CARTESIAN_POINT('Origin',(17.328,25.104,39.768));
#60041=CARTESIAN_POINT('Origin',(13.872,22.44,39.168));
#60042=CARTESIAN_POINT('',(13.872,25.104,20.196));
#60043=CARTESIAN_POINT('Origin',(14.472,25.104,20.196));
#60044=CARTESIAN_POINT('Origin',(13.872,22.44,48.552));
#60045=CARTESIAN_POINT('',(6.936,25.104,48.552));
#60046=CARTESIAN_POINT('Origin',(6.936,25.104,47.952));
#60047=CARTESIAN_POINT('Origin',(32.64,22.44,48.552));
#60048=CARTESIAN_POINT('Origin',(17.328,25.104,17.136));
#60049=CARTESIAN_POINT('Origin',(-8.1888,25.104,3.9984));
#60050=CARTESIAN_POINT('',(-7.5888,25.104,-21.7872));
#60051=CARTESIAN_POINT('',(-7.5888,25.104,3.9984));
#60052=CARTESIAN_POINT('Origin',(-8.1888,25.104,-21.7872));
#60053=CARTESIAN_POINT('Origin',(0.,25.104,-21.7872));
#60054=CARTESIAN_POINT('Origin',(0.,25.104,-21.7872));
#60055=CARTESIAN_POINT('Origin',(7.5888,22.44,-21.7872));
#60056=CARTESIAN_POINT('',(7.5888,22.44,-21.7872));
#60057=CARTESIAN_POINT('Origin',(0.,22.44,-21.7872));
#60058=CARTESIAN_POINT('',(-7.5888,22.44,-21.7872));
#60059=CARTESIAN_POINT('Origin',(-7.5888,22.44,6.7728));
#60060=CARTESIAN_POINT('Origin',(14.28,25.104,-35.688));
#60061=CARTESIAN_POINT('Origin',(17.952,25.104,-35.088));
#60062=CARTESIAN_POINT('Origin',(17.952,25.104,-35.088));
#60063=CARTESIAN_POINT('Origin',(17.352,25.104,-16.932));
#60064=CARTESIAN_POINT('',(17.952,25.104,-16.932));
#60065=CARTESIAN_POINT('Origin',(17.952,22.44,-35.088));
#60066=CARTESIAN_POINT('Origin',(17.952,22.44,-35.088));
#60067=CARTESIAN_POINT('Origin',(-28.152,25.104,28.56));
#60068=CARTESIAN_POINT('Origin',(-28.152,25.104,31.66));
#60069=CARTESIAN_POINT('Origin',(3.456,25.104,-17.136));
#60070=CARTESIAN_POINT('Origin',(3.456,25.104,-37.944));
#60071=CARTESIAN_POINT('Origin',(3.456,25.104,-35.496));
#60072=CARTESIAN_POINT('Origin',(0.,25.104,-35.496));
#60073=CARTESIAN_POINT('',(-2.856,25.104,-35.496));
#60074=CARTESIAN_POINT('Origin',(-3.456,25.104,-35.496));
#60075=CARTESIAN_POINT('Origin',(0.,25.104,-35.496));
#60076=CARTESIAN_POINT('Origin',(-3.456,25.104,-18.36));
#60077=CARTESIAN_POINT('Origin',(-3.456,25.104,-37.944));
#60078=CARTESIAN_POINT('',(-2.856,25.104,-18.36));
#60079=CARTESIAN_POINT('Origin',(0.,25.104,-37.944));
#60080=CARTESIAN_POINT('Origin',(0.,22.44,-35.496));
#60081=CARTESIAN_POINT('',(-2.856,22.44,-35.496));
#60082=CARTESIAN_POINT('Origin',(-29.376,25.104,38.352));
#60083=CARTESIAN_POINT('Origin',(-29.376,25.104,33.6154718625761));
#60084=CARTESIAN_POINT('Origin',(29.376,25.104,38.352));
#60085=CARTESIAN_POINT('',(25.0637359312881,25.5282640687119,38.352));
#60086=CARTESIAN_POINT('',(29.376,25.5282640687119,34.0397359312881));
#60087=CARTESIAN_POINT('Origin',(29.376,25.5282640687119,38.352));
#60088=CARTESIAN_POINT('Origin',(29.376,25.104,33.6154718625761));
#60089=CARTESIAN_POINT('Origin',(29.376,25.5282640687119,38.352));
#60090=CARTESIAN_POINT('Origin',(29.376,25.296,38.352));
#60091=CARTESIAN_POINT('',(29.376,25.0637359312881,42.1997359312881));
#60092=CARTESIAN_POINT('',(25.5282640687119,25.0637359312881,38.352));
#60093=CARTESIAN_POINT('Origin',(29.376,25.0637359312881,38.352));
#60094=CARTESIAN_POINT('Origin',(29.376,25.0637359312881,38.352));
#60095=CARTESIAN_POINT('',(25.296,25.296,38.352));
#60096=CARTESIAN_POINT('Origin',(29.376,24.6394718625761,38.352));
#60097=CARTESIAN_POINT('Origin',(29.376,24.6394718625761,42.624));
#60098=CARTESIAN_POINT('Origin',(-2.856,22.44,-37.944));
#60099=CARTESIAN_POINT('Origin',(-13.872,22.44,13.056));
#99994=UNCERTAINTY_MEASURE_WITH_UNIT(LENGTH_MEASURE(0.01),#100032,
'DISTANCE_ACCURACY_VALUE',
'Maximum model space distance between geometric entities at asserted c
onnectivities');
#100011=UNCERTAINTY_MEASURE_WITH_UNIT(LENGTH_MEASURE(0.01),#100032,
'DISTANCE_ACCURACY_VALUE',
'Maximum model space distance between geometric entities at asserted c
onnectivities');
#100014=(
GEOMETRIC_REPRESENTATION_CONTEXT(3)
GLOBAL_UNCERTAINTY_ASSIGNED_CONTEXT((#99994))
GLOBAL_UNIT_ASSIGNED_CONTEXT((#100032,#100034,#100035))
REPRESENTATION_CONTEXT('','3D')
);
#100031=(
GEOMETRIC_REPRESENTATION_CONTEXT(3)
GLOBAL_UNCERTAINTY_ASSIGNED_CONTEXT((#100011))
GLOBAL_UNIT_ASSIGNED_CONTEXT((#100032,#100034,#100035))
REPRESENTATION_CONTEXT('','3D')
);
#100032=(
LENGTH_UNIT()
NAMED_UNIT(*)
SI_UNIT(.MILLI.,.METRE.)
);
#100034=(
NAMED_UNIT(*)
PLANE_ANGLE_UNIT()
SI_UNIT($,.RADIAN.)
);
#100035=(
NAMED_UNIT(*)
SI_UNIT($,.STERADIAN.)
SOLID_ANGLE_UNIT()
);
#100038=SHAPE_DEFINITION_REPRESENTATION(#100057,#100102);
#100057=PRODUCT_DEFINITION_SHAPE('',$,#100122);
#100102=SHAPE_REPRESENTATION('',(#20343),#100014);
#100119=PRODUCT_DEFINITION_CONTEXT('part definition',#100178,'design');
#100122=PRODUCT_DEFINITION('2026-10-12-11-54-52-874',
'02_Actuator_Frame_Plate',#100141,#100119);
#100141=PRODUCT_DEFINITION_FORMATION('',$,#100182);
#100178=APPLICATION_CONTEXT(
'Core Data for Automotive Mechanical Design Process');
#100179=PRODUCT_CONTEXT('part definition',#100178,'mechanical');
#100182=PRODUCT('2026-10-12-11-54-52-874','02_Actuator_Frame_Plate',$,(#100179));
#100201=PRESENTATION_STYLE_ASSIGNMENT((#100207));
#100207=SURFACE_STYLE_USAGE(.BOTH.,#100213);
#100213=SURFACE_SIDE_STYLE('',(#100219));
#100219=SURFACE_STYLE_FILL_AREA(#100225);
#100225=FILL_AREA_STYLE('Opaque(20,51,87)',(#100231));
#100231=FILL_AREA_STYLE_COLOUR('Opaque(20,51,87)',#100237);
#100237=COLOUR_RGB('Opaque(20,51,87)',0.0784313725490196,0.2,0.341176470588235);
ENDSEC;
END-ISO-10303-21;
